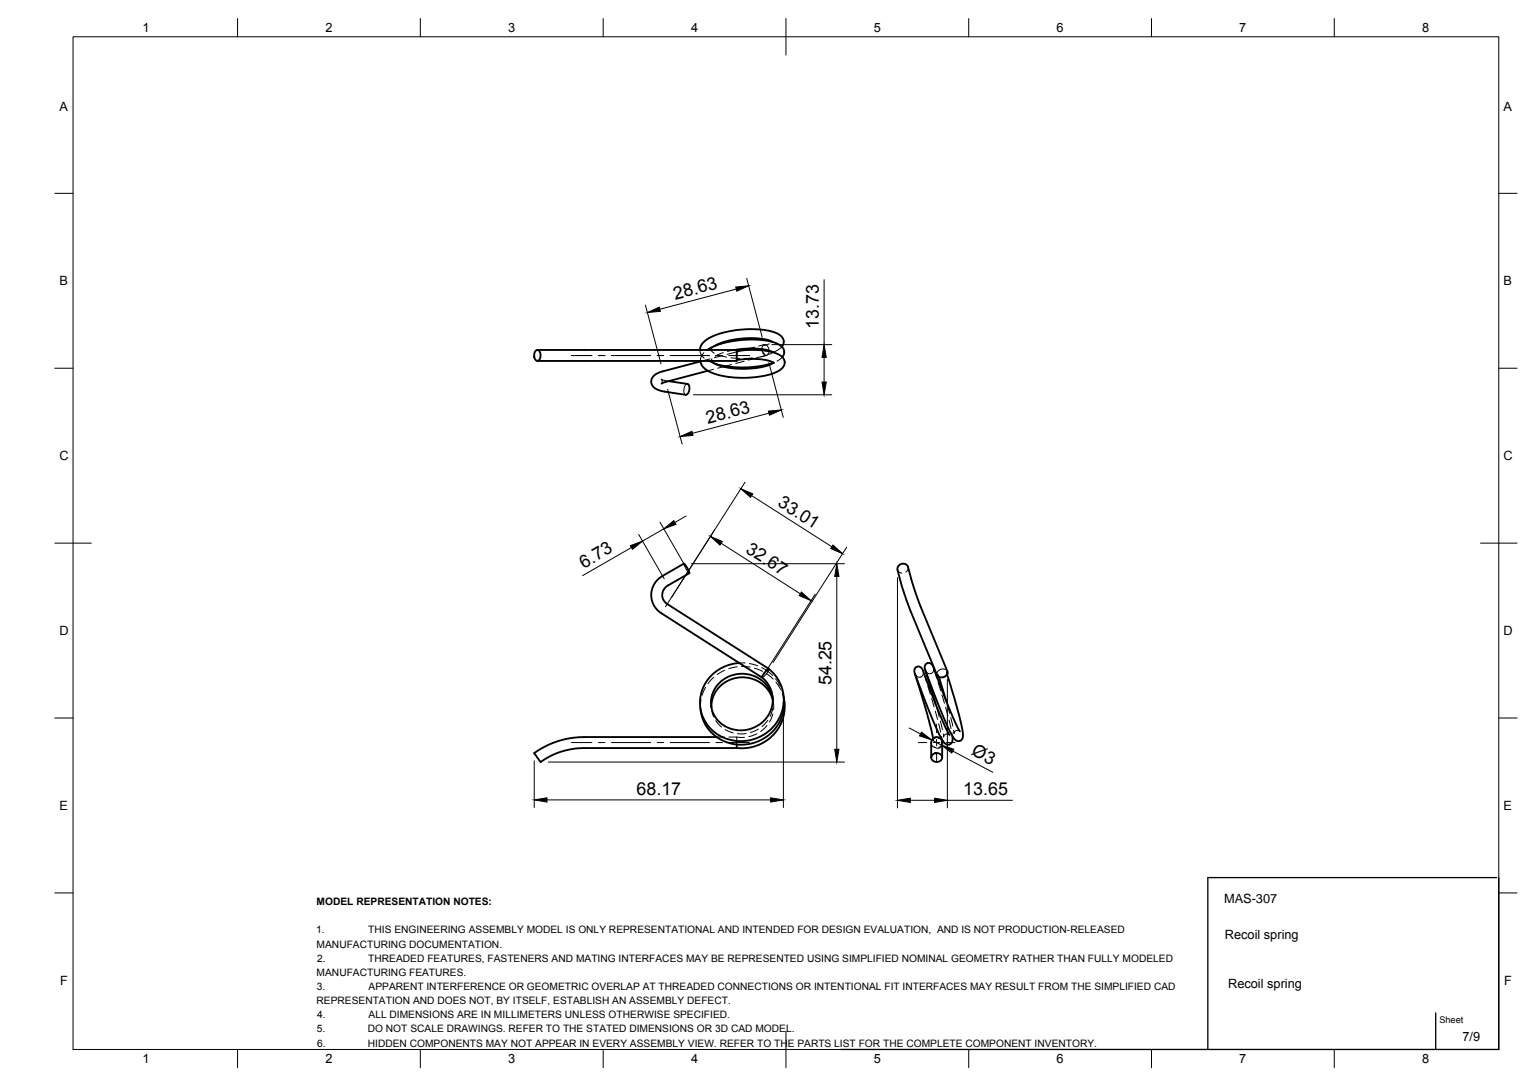
ISO-10303-21;
HEADER;
FILE_DESCRIPTION (('STEP AP214'),
    '1' );
FILE_NAME ('Recoil spring.step',
    '2026-10-06T07:34:29',
    ( '' ),
    ( '' ),
    'SwSTEP 2.0',
    'SolidWorks 2025',
    '' );
FILE_SCHEMA (( 'AUTOMOTIVE_DESIGN' ));
ENDSEC;

DATA;
#11=CARTESIAN_POINT ( 'NONE',  ( 205.4931693814993139, 33.91842896272902408, -6.501828201457912293 ) ) ;
#21=CARTESIAN_POINT ( 'NONE',  ( 205.4699394944333051, 33.88363592193200446, -7.930995773285529182 ) ) ;
#30=CARTESIAN_POINT ( 'NONE',  ( 198.8634854004546071, 49.55149448133588663, -6.680369717582868461 ) ) ;
#56=TOROIDAL_SURFACE ( 'NONE', #1821, 4.799128011492294732, 1.499999999999997113 ) ;
#64=CARTESIAN_POINT ( 'NONE',  ( 207.1592428330643827, 35.64176030267155681, -3.375779224823745928 ) ) ;
#71=CARTESIAN_POINT ( 'NONE',  ( 198.4684236769687686, 29.09143143995051872, -2.316743362709667409 ) ) ;
#88=CARTESIAN_POINT ( 'NONE',  ( 198.7876695280922661, 49.53587328158837977, -8.249370650301745655 ) ) ;
#95=CARTESIAN_POINT ( 'NONE',  ( 201.7406124912899941, 52.65652330452660834, -2.244206067705167396 ) ) ;
#103=CARTESIAN_POINT ( 'NONE',  ( 202.3883256910358739, 32.65987148549056229, -8.116337980372584582 ) ) ;
#123=DIRECTION ( 'NONE',  ( -0.9741547192086867923, 0.2258817899775114602, 0.000000000000000000 ) ) ;
#132=CARTESIAN_POINT ( 'NONE',  ( 202.9578473199472057, 32.84482942423175444, -9.656098271102047548 ) ) ;
#152=FACE_OUTER_BOUND ( 'NONE', #9575, .T. ) ;
#166=CARTESIAN_POINT ( 'NONE',  ( 198.3913412372077687, 29.09831693401786268, -0.7477385443502184703 ) ) ;
#174=CARTESIAN_POINT ( 'NONE',  ( 207.1690005588685040, 46.08364065960329725, 0.3832845883476674320 ) ) ;
#205=CARTESIAN_POINT ( 'NONE',  ( 205.4339596421060889, 33.86846485884471747, -4.932823326473320336 ) ) ;
#208=CIRCLE ( 'NONE', #2252, 1.499999999999996891 ) ;
#212=CARTESIAN_POINT ( 'NONE',  ( 192.9105869384611935, 31.39693960586098598, -5.567602151433582058 ) ) ;
#219=AXIS2_PLACEMENT_3D ( 'NONE', #7961, #12749, #6770 ) ;
#229=EDGE_CURVE ( 'NONE', #11059, #5257, #8156, .T. ) ;
#231=DIRECTION ( 'NONE',  ( 0.9296197478520974444, 0.3660421972118351741, -0.04266420354037655377 ) ) ;
#237=CARTESIAN_POINT ( 'NONE',  ( 207.1194509196011495, 46.14302886020001182, -1.185720282267065828 ) ) ;
#249=CARTESIAN_POINT ( 'NONE',  ( 194.7047954745769687, 33.92018974228710704, -0.9908858387024377379 ) ) ;
#258=CARTESIAN_POINT ( 'NONE',  ( 202.9147226314038051, 48.88641379461363101, -0.9068510277452211943 ) ) ;
#277=ORIENTED_EDGE ( 'NONE', *, *, #6163, .F. ) ;
#281=DIRECTION ( 'NONE',  ( -0.9741547192086869034, 0.2258817899775114879, 0.000000000000000000 ) ) ;
#291=CARTESIAN_POINT ( 'NONE',  ( 191.3844089520862894, 42.02011290432638901, -3.056456915890917170 ) ) ;
#298=CARTESIAN_POINT ( 'NONE',  ( 204.3096479244403554, 51.57035008254927533, -0.9325724660367167296 ) ) ;
#317=CARTESIAN_POINT ( 'NONE',  ( 207.1167095084715868, 46.15093117762712893, -7.185265714380067337 ) ) ;
#325=CARTESIAN_POINT ( 'NONE',  ( 203.1202131991386182, 29.73909689272393564, -6.555651296533415717 ) ) ;
#329=TOROIDAL_SURFACE ( 'NONE', #6419, 4.799128011492294732, 1.499999999999997113 ) ;
#334=CARTESIAN_POINT ( 'NONE',  ( 198.9393012728169765, 49.56711568108339350, -5.111368784863990378 ) ) ;
#366=CARTESIAN_POINT ( 'NONE',  ( 194.7957337413261030, 33.86335648926068842, -5.558215102112974648 ) ) ;
#393=CARTESIAN_POINT ( 'NONE',  ( 198.8872864542346974, 32.16591232847088122, -2.310211674251309688 ) ) ;
#410=CARTESIAN_POINT ( 'NONE',  ( 194.8975446553719451, 47.93174114899129989, -1.867390259657528251 ) ) ;
#442=CARTESIAN_POINT ( 'NONE',  ( 208.8124460758720033, 42.05191026284237665, -4.433604294307299298 ) ) ;
#471=CARTESIAN_POINT ( 'NONE',  ( 198.8863654052626657, 49.55881746625484396, -3.681704842056328086 ) ) ;
#489=CARTESIAN_POINT ( 'NONE',  ( 201.2644297667355886, 32.15691159195442594, -0.6119088838163699862 ) ) ;
#491=ADVANCED_FACE ( 'NONE', ( #11969 ), #1138, .F. ) ;
#494=DIRECTION ( 'NONE',  ( 0.000000000000000000, 0.9569673715906176215, 0.2901955370279575286 ) ) ;
#525=CARTESIAN_POINT ( 'NONE',  ( 207.1194509196011495, 46.14302886020001182, -1.185720282267065828 ) ) ;
#557=CARTESIAN_POINT ( 'NONE',  ( 205.4319281802536068, 33.87189768065903905, -1.932853472788024440 ) ) ;
#566=CARTESIAN_POINT ( 'NONE',  ( 202.1731860119849102, 31.08132011834958419, -8.150590381057213563 ) ) ;
#575=CARTESIAN_POINT ( 'NONE',  ( 207.3546231538492179, 50.29643094772573164, -2.498001438440778710 ) ) ;
#577=EDGE_LOOP ( 'NONE', ( #6152, #5245, #8146, #7504 ) ) ;
#580=LINE ( 'NONE', #12899, #7977 ) ;
#623=CARTESIAN_POINT ( 'NONE',  ( 203.1375244286944906, 48.81137831324044640, 0.6531691591918254991 ) ) ;
#642=MANIFOLD_SOLID_BREP ( 'Sweep1', #13662 ) ;
#651=CARTESIAN_POINT ( 'NONE',  ( 211.8663679066739007, 39.14335912920272875, 0.001962313962203070510 ) ) ;
#654=CARTESIAN_POINT ( 'NONE',  ( 166.7445055987502656, 66.43865443379107205, -0.9107274384406879308 ) ) ;
#688=DIRECTION ( 'NONE',  ( 0.6130913241491352528, 0.7900120431063440973, -6.390853288732736916E-17 ) ) ;
#690=PRODUCT ( 'Recoil spring', 'Recoil spring', '', ( #15067 ) ) ;
#693=FACE_OUTER_BOUND ( 'NONE', #15416, .T. ) ;
#706=DIRECTION ( 'NONE',  ( -1.000000000000000000, 0.000000000000000000, 0.000000000000000000 ) ) ;
#709=CARTESIAN_POINT ( 'NONE',  ( 205.5168546899054434, 47.82311440310952833, -1.064259200291542529 ) ) ;
#724=EDGE_LOOP ( 'NONE', ( #6088, #7663, #14419, #15071, #11022 ) ) ;
#727=CARTESIAN_POINT ( 'NONE',  ( 201.6516474359912934, 52.64960446646696113, -8.385050746608255778 ) ) ;
#736=VECTOR ( 'NONE', #8355, 999.9999999999998863 ) ;
#780=CARTESIAN_POINT ( 'NONE',  ( 207.3736904795575811, 50.31851200600168994, -2.642755332960478043 ) ) ;
#790=DIRECTION ( 'NONE',  ( -1.000000000000000000, 0.000000000000000000, 0.000000000000000000 ) ) ;
#809=CARTESIAN_POINT ( 'NONE',  ( 188.2965488188713721, 39.35787245461563089, -4.374714073396582137 ) ) ;
#863=CARTESIAN_POINT ( 'NONE',  ( 198.5781842723177704, 29.07471546161169229, -6.884323831650920766 ) ) ;
#870=DIRECTION ( 'NONE',  ( 0.000000000000000000, 0.000000000000000000, -1.000000000000000000 ) ) ;
#887=CARTESIAN_POINT ( 'NONE',  ( 190.6753907620029054, 48.10438271498464502, -4.747728522856008659 ) ) ;
#898=CARTESIAN_POINT ( 'NONE',  ( 208.8119045081773777, 39.60750423734790360, -5.989029428842635561 ) ) ;
#906=TOROIDAL_SURFACE ( 'NONE', #7237, 21.91351791792154202, 1.499999999999997113 ) ;
#965=CARTESIAN_POINT ( 'NONE',  ( 198.8104769829885754, 49.54338459298288200, -5.250705761417654216 ) ) ;
#975=CARTESIAN_POINT ( 'NONE',  ( 198.8872864542346974, 32.16591232847088122, -2.310211674251309688 ) ) ;
#982=CIRCLE ( 'NONE', #8569, 1.499999999999994227 ) ;
#983=CARTESIAN_POINT ( 'NONE',  ( 208.8060099514817978, 42.07246638764446089, -7.432400171711813996 ) ) ;
#996=DIRECTION ( 'NONE',  ( 0.000000000000000000, 0.000000000000000000, -1.000000000000000000 ) ) ;
#1021=CARTESIAN_POINT ( 'NONE',  ( 192.9079700310636269, 50.30505391962363149, -5.011923969639807019 ) ) ;
#1022=PRESENTATION_STYLE_ASSIGNMENT (( #8312 ) ) ;
#1052=CARTESIAN_POINT ( 'NONE',  ( 207.1558710170397433, 35.63411313097393673, -9.376170956558697256 ) ) ;
#1063=CARTESIAN_POINT ( 'NONE',  ( 201.2541767070109984, 32.14103196098812987, -5.186035738131804962 ) ) ;
#1081=FACE_OUTER_BOUND ( 'NONE', #6812, .T. ) ;
#1088=SHAPE_REPRESENTATION_RELATIONSHIP ( 'NONE' , 'NONE' ,  #5419, #10743 ) ;
#1097=EDGE_CURVE ( 'NONE', #8873, #8651, #1552, .T. ) ;
#1100=CARTESIAN_POINT ( 'NONE',  ( 208.8060099514817978, 42.07246638764446089, -7.432400171711813996 ) ) ;
#1102=EDGE_LOOP ( 'NONE', ( #10073, #2655 ) ) ;
#1128=CARTESIAN_POINT ( 'NONE',  ( 211.8745662956760896, 42.53653439883859022, -6.011979689023970508 ) ) ;
#1130=CARTESIAN_POINT ( 'NONE',  ( 166.9217645774054120, 62.57671370024034729, -0.9107274384406883749 ) ) ;
#1136=CARTESIAN_POINT ( 'NONE',  ( 198.8634854004546071, 49.55149448133588663, -6.680369717582868461 ) ) ;
#1138=PLANE ( 'NONE',  #4834 ) ;
#1145=CARTESIAN_POINT ( 'NONE',  ( 208.8051451104704768, 39.65587490144260840, -4.559632177755815086 ) ) ;
#1172=CARTESIAN_POINT ( 'NONE',  ( 205.4931693814993139, 33.91842896272902408, -6.501828201457912293 ) ) ;
#1186=ORIENTED_EDGE ( 'NONE', *, *, #3880, .F. ) ;
#1195=CARTESIAN_POINT ( 'NONE',  ( 211.8802283582561472, 39.29745248741442509, -3.136047433260559902 ) ) ;
#1208=CARTESIAN_POINT ( 'NONE',  ( 198.8863654052626657, 49.55881746625484396, -3.681704842056328086 ) ) ;
#1216=CARTESIAN_POINT ( 'NONE',  ( 201.2541767070109984, 32.14103196098812987, -5.186035738131804962 ) ) ;
#1231=DIRECTION ( 'NONE',  ( -0.2258817899775119320, -0.9741547192086866813, 0.000000000000000000 ) ) ;
#1255=CARTESIAN_POINT ( 'NONE',  ( 198.9643688939780191, 32.15902683440354082, -3.879216492611309519 ) ) ;
#1261=CARTESIAN_POINT ( 'NONE',  ( 192.9009781015629699, 50.32399521507879570, -6.439879401016198379 ) ) ;
#1282=CARTESIAN_POINT ( 'NONE',  ( 201.1886137893777970, 49.58779752487713210, -5.375724496774349603 ) ) ;
#1290=EDGE_CURVE ( 'NONE', #2155, #10688, #5789, .T. ) ;
#1291=CARTESIAN_POINT ( 'NONE',  ( 209.6520103264654438, 47.93571987055528183, -2.624305162434556582 ) ) ;
#1292=ORIENTED_EDGE ( 'NONE', *, *, #10887, .T. ) ;
#1320=ORIENTED_EDGE ( 'NONE', *, *, #15180, .T. ) ;
#1331=CARTESIAN_POINT ( 'NONE',  ( 208.8253499713366352, 39.76173270276598970, -9.127040822819912691 ) ) ;
#1356=CARTESIAN_POINT ( 'NONE',  ( 205.5168546899054434, 47.82311440310952833, -1.064259200291542529 ) ) ;
#1366=CARTESIAN_POINT ( 'NONE',  ( 190.5757627275658876, 33.76246512414177658, -1.122914728280356433 ) ) ;
#1371=CARTESIAN_POINT ( 'NONE',  ( 170.6931741512129577, -3.595212766542494887, -13.46247879130521952 ) ) ;
#1374=CARTESIAN_POINT ( 'NONE',  ( 201.3430548014149792, 49.57506994421799362, -2.237714600605053228 ) ) ;
#1386=CARTESIAN_POINT ( 'NONE',  ( 169.1145417280692698, 64.59938046134368506, -0.9107274384406877088 ) ) ;
#1392=LINE ( 'NONE', #3931, #8028 ) ;
#1403=EDGE_CURVE ( 'NONE', #5373, #11059, #4546, .T. ) ;
#1406=CARTESIAN_POINT ( 'NONE',  ( 194.7298858349713271, 47.80990288192585780, -8.002378029496236778 ) ) ;
#1413=CARTESIAN_POINT ( 'NONE',  ( 209.5813200025016840, 33.68906342850529256, -7.816773541869418196 ) ) ;
#1415=EDGE_CURVE ( 'NONE', #11153, #5773, #6043, .T. ) ;
#1421=ORIENTED_EDGE ( 'NONE', *, *, #1403, .T. ) ;
#1433=CARTESIAN_POINT ( 'NONE',  ( 193.1265229109121435, 35.50728864820005981, -5.680987958736793075 ) ) ;
#1439=CARTESIAN_POINT ( 'NONE',  ( 191.3907470605235801, 42.09736693221333326, -1.487451979171016125 ) ) ;
#1449=CARTESIAN_POINT ( 'NONE',  ( 205.4081958545874613, 47.87064854543508829, -4.057643371672452481 ) ) ;
#1485=CARTESIAN_POINT ( 'NONE',  ( 191.3918663844754349, 39.68659111044760124, -5.934329888686073140 ) ) ;
#1493=CARTESIAN_POINT ( 'NONE',  ( 190.6654829352982290, 48.12161981134465805, -3.320406740534335377 ) ) ;
#1517=CARTESIAN_POINT ( 'NONE',  ( 207.1288103955774318, 46.12660085639766550, -4.186765234109192768 ) ) ;
#1527=CARTESIAN_POINT ( 'NONE',  ( 188.2965488188713721, 39.35787245461563089, -4.374714073396582137 ) ) ;
#1535=CARTESIAN_POINT ( 'NONE',  ( 198.9622538275367845, 49.57425033952682014, -2.112703922695001513 ) ) ;
#1552=LINE ( 'NONE', #13232, #4560 ) ;
#1595=CARTESIAN_POINT ( 'NONE',  ( 191.3844089520862894, 42.02011290432638901, -3.056456915890917170 ) ) ;
#1603=EDGE_CURVE ( 'NONE', #11059, #9376, #6576, .T. ) ;
#1618=CARTESIAN_POINT ( 'NONE',  ( 191.3767946852191528, 39.76267059705192253, -4.365329018565075714 ) ) ;
#1675=CARTESIAN_POINT ( 'NONE',  ( 198.8863654052626657, 49.55881746625484396, -3.681704842056328086 ) ) ;
#1676=ORIENTED_EDGE ( 'NONE', *, *, #12956, .T. ) ;
#1685=DIRECTION ( 'NONE',  ( -0.8204839007831801201, 0.5707893219124390294, -0.03171306586179811760 ) ) ;
#1692=CARTESIAN_POINT ( 'NONE',  ( 194.7047954745769687, 33.92018974228710704, -0.9908858387024377379 ) ) ;
#1740=ORIENTED_EDGE ( 'NONE', *, *, #9984, .T. ) ;
#1752=CARTESIAN_POINT ( 'NONE',  ( 193.1249951165660548, 46.22013307728793308, -3.310989833511668756 ) ) ;
#1754=DIRECTION ( 'NONE',  ( -0.2258817899775119320, -0.9741547192086866813, 0.000000000000000000 ) ) ;
#1771=CARTESIAN_POINT ( 'NONE',  ( 207.2666510146856069, 31.35441966018789728, -3.370316356820458381 ) ) ;
#1803=CARTESIAN_POINT ( 'NONE',  ( 191.4227524587821279, 39.61567282607229856, -2.929995994935606252 ) ) ;
#1810=DIRECTION ( 'NONE',  ( -0.7900120431063429871, 0.6130913241491365850, 0.000000000000000000 ) ) ;
#1811=CARTESIAN_POINT ( 'NONE',  ( 173.2749560924322907, 69.96037208313981637, -0.9107274384406881529 ) ) ;
#1818=CARTESIAN_POINT ( 'NONE',  ( 207.3157014670556748, 31.37515976295564357, -6.367693553816072161 ) ) ;
#1821=AXIS2_PLACEMENT_3D ( 'NONE', #5536, #6883, #15294 ) ;
#1844=CARTESIAN_POINT ( 'NONE',  ( 198.4239224672526234, 29.08807987246144933, -3.746314016867685837 ) ) ;
#1851=DIRECTION ( 'NONE',  ( 0.000000000000000000, 0.9569673715906176215, 0.2901955370279575286 ) ) ;
#1892=CARTESIAN_POINT ( 'NONE',  ( 201.6895650671498288, 29.08490409614774208, -0.6212496039192949571 ) ) ;
#1901=EDGE_LOOP ( 'NONE', ( #1292, #1740, #6793, #7476 ) ) ;
#1906=CARTESIAN_POINT ( 'NONE',  ( 205.4339596421060889, 33.86846485884471747, -4.932823326473320336 ) ) ;
#1921=CARTESIAN_POINT ( 'NONE',  ( 209.6393851568315938, 47.95822392590527983, 0.3767681043515945238 ) ) ;
#1957=FACE_OUTER_BOUND ( 'NONE', #577, .T. ) ;
#1960=LINE ( 'NONE', #6798, #8102 ) ;
#1970=CARTESIAN_POINT ( 'NONE',  ( 207.2819921120892275, 50.35227183911742088, -8.638656677529437999 ) ) ;
#1979=DIRECTION ( 'NONE',  ( 0.000000000000000000, 0.000000000000000000, -1.000000000000000000 ) ) ;
#1999=CARTESIAN_POINT ( 'NONE',  ( 198.5423134874356208, 52.64753739496011065, -2.122073255223759780 ) ) ;
#2041=DIRECTION ( 'NONE',  ( 0.000000000000000000, 0.000000000000000000, -1.000000000000000000 ) ) ;
#2050=CARTESIAN_POINT ( 'NONE',  ( 207.5020891771285960, 50.23084475345794431, 0.4952462535581279024 ) ) ;
#2080=CARTESIAN_POINT ( 'NONE',  ( 207.2638851143210275, 31.35908548908414417, -0.3703513705075706097 ) ) ;
#2130=CARTESIAN_POINT ( 'NONE',  ( 188.3492591927541753, 42.47468418338397811, -7.638025320682917396 ) ) ;
#2146=ORIENTED_EDGE ( 'NONE', *, *, #4376, .F. ) ;
#2155=VERTEX_POINT ( 'NONE', #1811 ) ;
#2157=CARTESIAN_POINT ( 'NONE',  ( 194.7298858349713271, 47.80990288192585780, -8.002378029496236778 ) ) ;
#2170=CARTESIAN_POINT ( 'NONE',  ( 191.4249991583111523, 42.11970308376083949, -6.062475933048471433 ) ) ;
#2211=CARTESIAN_POINT ( 'NONE',  ( 203.2625657313046190, 29.78760669494945645, -9.693656633365744568 ) ) ;
#2236=CARTESIAN_POINT ( 'NONE',  ( 193.0816233526163046, 46.15577860858359571, -4.879990690958216248 ) ) ;
#2248=CARTESIAN_POINT ( 'NONE',  ( 207.0703735592109069, 35.50494473061488065, -6.238171316985951620 ) ) ;
#2252=AXIS2_PLACEMENT_3D ( 'NONE', #1130, #15560, #8420 ) ;
#2256=CARTESIAN_POINT ( 'NONE',  ( 198.9111841706756536, 32.15857605477618364, -5.308824953579920347 ) ) ;
#2277=CIRCLE ( 'NONE', #12605, 23.41351791792154202 ) ;
#2280=CARTESIAN_POINT ( 'NONE',  ( 202.9928097691983169, 48.86380790798758511, -0.9029304599467440351 ) ) ;
#2291=CARTESIAN_POINT ( 'NONE',  ( 205.4699394944333051, 33.88363592193200446, -7.930995773285529182 ) ) ;
#2301=ORIENTED_EDGE ( 'NONE', *, *, #12956, .F. ) ;
#2321=CARTESIAN_POINT ( 'NONE',  ( 193.1767286061335653, 35.44822858574072910, -7.249992917093472933 ) ) ;
#2332=CARTESIAN_POINT ( 'NONE',  ( 191.3918663844754349, 39.68659111044760124, -5.934329888686073140 ) ) ;
#2341=CARTESIAN_POINT ( 'NONE',  ( 207.1131222881253393, 35.56952893079440514, -7.807171136772324438 ) ) ;
#2370=CARTESIAN_POINT ( 'NONE',  ( 207.1558710170397433, 35.63411313097393673, -9.376170956558697256 ) ) ;
#2388=EDGE_CURVE ( 'NONE', #6288, #10688, #1960, .T. ) ;
#2397=CARTESIAN_POINT ( 'NONE',  ( 198.3905366428873549, 52.61667164843417765, -5.260075093946414704 ) ) ;
#2406=CARTESIAN_POINT ( 'NONE',  ( 201.3402840685550643, 32.17245832385849980, -2.180909807981465054 ) ) ;
#2447=CARTESIAN_POINT ( 'NONE',  ( 205.5291621427655002, 33.93354315402728361, -9.500001906449378808 ) ) ;
#2470=CARTESIAN_POINT ( 'NONE',  ( 205.4911088677281725, 33.92184391926740972, -3.501858402168778639 ) ) ;
#2484=CARTESIAN_POINT ( 'NONE',  ( 198.4239224672526234, 29.08807987246144933, -3.746314016867685837 ) ) ;
#2489=DIRECTION ( 'NONE',  ( -0.1562424607007877608, 0.2866315678550999668, -0.9452145987991775744 ) ) ;
#2528=CARTESIAN_POINT ( 'NONE',  ( 202.4595012533446550, 32.68412682837883665, -9.685340726858029825 ) ) ;
#2535=CARTESIAN_POINT ( 'NONE',  ( 209.5863484626195543, 33.70058422559537092, -1.816147585399736863 ) ) ;
#2552=CIRCLE ( 'NONE', #3062, 3.299128011492291623 ) ;
#2566=CARTESIAN_POINT ( 'NONE',  ( 190.7088546992480076, 48.18597428004899541, -1.751405883087224113 ) ) ;
#2608=CARTESIAN_POINT ( 'NONE',  ( 202.3883256910358739, 32.65987148549056229, -8.116337980372584582 ) ) ;
#2635=CARTESIAN_POINT ( 'NONE',  ( 194.7691866843436799, 33.87697957786221536, -2.559886773443665220 ) ) ;
#2645=CARTESIAN_POINT ( 'NONE',  ( 198.5110307061451067, 52.63772278181842523, -5.120705508804510586 ) ) ;
#2653=CARTESIAN_POINT ( 'NONE',  ( 203.1375244286944906, 48.81137831324044640, 0.6531691591918254991 ) ) ;
#2655=ORIENTED_EDGE ( 'NONE', *, *, #1415, .F. ) ;
#2712=CARTESIAN_POINT ( 'NONE',  ( 208.8124460758720033, 42.05191026284237665, -4.433604294307299298 ) ) ;
#2720=CARTESIAN_POINT ( 'NONE',  ( 193.1683668805158334, 46.28448754599228465, -1.741988976065122152 ) ) ;
#2730=CARTESIAN_POINT ( 'NONE',  ( 191.4227524587821279, 39.61567282607229856, -2.929995994935606252 ) ) ;
#2773=CARTESIAN_POINT ( 'NONE',  ( 188.3535365708562779, 39.18556319200014570, -2.939344140512093251 ) ) ;
#2774=CIRCLE ( 'NONE', #11846, 1.499999999999988232 ) ;
#2780=ORIENTED_EDGE ( 'NONE', *, *, #4665, .F. ) ;
#2785=CYLINDRICAL_SURFACE ( 'NONE', #15558, 1.500000000000000444 ) ;
#2792=LINE ( 'NONE', #7617, #5517 ) ;
#2793=CARTESIAN_POINT ( 'NONE',  ( 202.9147226314038051, 48.88641379461363101, -0.9068510277452211943 ) ) ;
#2813=CARTESIAN_POINT ( 'NONE',  ( 202.8187013049204950, 32.78779105710274422, -6.518094968334741779 ) ) ;
#2852=CARTESIAN_POINT ( 'NONE',  ( 209.6082252582704371, 33.74895655718308518, -4.813932606105665535 ) ) ;
#2869=FACE_OUTER_BOUND ( 'NONE', #5166, .T. ) ;
#2873=CARTESIAN_POINT ( 'NONE',  ( 203.1427736312160164, 48.80054947466439330, -2.493724563924679671 ) ) ;
#2884=ORIENTED_EDGE ( 'NONE', *, *, #4665, .T. ) ;
#2892=CARTESIAN_POINT ( 'NONE',  ( 208.8213467238098247, 41.99652926550911758, -5.863399402755005596 ) ) ;
#2909=AXIS2_PLACEMENT_3D ( 'NONE', #7942, #5322, #5486 ) ;
#2923=CARTESIAN_POINT ( 'NONE',  ( 208.8002188652075972, 39.64064887424692785, -1.560527519332197022 ) ) ;
#2964=UNCERTAINTY_MEASURE_WITH_UNIT (LENGTH_MEASURE( 1.000000000000000082E-05 ), #13235, 'distance_accuracy_value', 'NONE');
#2965=CARTESIAN_POINT ( 'NONE',  ( 208.8276044750562335, 41.97590694738037342, -2.864603354092789100 ) ) ;
#2997=CARTESIAN_POINT ( 'NONE',  ( 194.7891036845171300, 47.85977741052224133, -6.433373108600371815 ) ) ;
#3015=CARTESIAN_POINT ( 'NONE',  ( 192.9601959511087728, 50.37386974367067438, -4.870874480120333416 ) ) ;
#3027=CARTESIAN_POINT ( 'NONE',  ( 205.4496313998743915, 47.84832575209421890, -7.060263518810960370 ) ) ;
#3045=CARTESIAN_POINT ( 'NONE',  ( 202.5558682508970492, 29.63341987102701580, -9.723657537314917221 ) ) ;
#3046=ORIENTED_EDGE ( 'NONE', *, *, #1403, .F. ) ;
#3054=ADVANCED_FACE ( 'NONE', ( #9769 ), #906, .T. ) ;
#3062=AXIS2_PLACEMENT_3D ( 'NONE', #5627, #1979, #706 ) ;
#3094=CARTESIAN_POINT ( 'NONE',  ( 204.3809113867051508, 51.54681031777401756, 0.6364305089822913652 ) ) ;
#3112=ORIENTED_EDGE ( 'NONE', *, *, #6453, .T. ) ;
#3118=CARTESIAN_POINT ( 'NONE',  ( 192.8103048780560584, 31.45858264101640600, -1.000270116828862133 ) ) ;
#3165=CARTESIAN_POINT ( 'NONE',  ( 198.3905366428873549, 52.61667164843417765, -5.260075093946414704 ) ) ;
#3176=CARTESIAN_POINT ( 'NONE',  ( 208.8162124854775357, 42.04914431719598156, -1.433821094984975009 ) ) ;
#3183=EDGE_CURVE ( 'NONE', #10985, #5154, #580, .T. ) ;
#3189=DIRECTION ( 'NONE',  ( -0.9429519417310716634, 0.3294944882152614496, 0.04769714688914629408 ) ) ;
#3192=CARTESIAN_POINT ( 'NONE',  ( 198.5781842723177704, 29.07471546161169229, -6.884323831650920766 ) ) ;
#3227=CARTESIAN_POINT ( 'NONE',  ( 172.0899380277727744, 70.88000906936352408, -0.9107274384406883749 ) ) ;
#3236=ORIENTED_EDGE ( 'NONE', *, *, #1603, .T. ) ;
#3238=CARTESIAN_POINT ( 'NONE',  ( 207.2638851143210275, 31.35908548908414417, -0.3703513705075706097 ) ) ;
#3270=CARTESIAN_POINT ( 'NONE',  ( 207.3157014670556748, 31.37515976295564357, -6.367693553816072161 ) ) ;
#3322=CARTESIAN_POINT ( 'NONE',  ( 211.8657363685815653, 42.56416725473636831, -9.010781945348840694 ) ) ;
#3350=CARTESIAN_POINT ( 'NONE',  ( 198.5455061167297117, 29.08454594588317477, -3.885748181069116569 ) ) ;
#3358=AXIS2_PLACEMENT_3D ( 'NONE', #4025, #688, #1810 ) ;
#3361=CARTESIAN_POINT ( 'NONE',  ( 208.8213467238098247, 41.99652926550911758, -5.863399402755005596 ) ) ;
#3400=CARTESIAN_POINT ( 'NONE',  ( 192.9750851430037528, 31.35397111148814631, -7.136603044727629630 ) ) ;
#3427=CARTESIAN_POINT ( 'NONE',  ( 208.7906731791537425, 42.14840350977979710, -9.001400940668622397 ) ) ;
#3436=CARTESIAN_POINT ( 'NONE',  ( 208.8051451104704768, 39.65587490144260840, -4.559632177755815086 ) ) ;
#3446=CARTESIAN_POINT ( 'NONE',  ( 205.4496313998743915, 47.84832575209421890, -7.060263518810960370 ) ) ;
#3450=CARTESIAN_POINT ( 'NONE',  ( 202.3883256910358739, 32.65987148549056229, -8.116337980372584582 ) ) ;
#3473=CARTESIAN_POINT ( 'NONE',  ( 201.4161383703745400, 32.18800505576257365, -3.749910732146560122 ) ) ;
#3501=CARTESIAN_POINT ( 'NONE',  ( 201.8412736707888087, 29.11599755995149152, -3.759251452247287517 ) ) ;
#3512=CARTESIAN_POINT ( 'NONE',  ( 202.3883256910358739, 32.65987148549056229, -8.116337980372584582 ) ) ;
#3518=CARTESIAN_POINT ( 'NONE',  ( 203.7481738146713326, 51.76374178194004827, -0.9107274384406881529 ) ) ;
#3521=APPLICATION_CONTEXT ( 'automotive_design' ) ;
#3555=CARTESIAN_POINT ( 'NONE',  ( 205.4496313998743915, 47.84832575209421890, -7.060263518810960370 ) ) ;
#3569=COLOUR_RGB ( '', 0.40784314, 0.44705882, 0.49803922) ;
#3583=CARTESIAN_POINT ( 'NONE',  ( 209.5402858782260864, 48.07700032709870896, -2.761241636875660710 ) ) ;
#3593=CARTESIAN_POINT ( 'NONE',  ( 201.8629198063431716, 32.54887535240757757, -8.146526315903498627 ) ) ;
#3602=FACE_OUTER_BOUND ( 'NONE', #11632, .T. ) ;
#3623=DIRECTION ( 'NONE',  ( -1.000000000000000000, 0.000000000000000000, 0.000000000000000000 ) ) ;
#3634=AXIS2_PLACEMENT_3D ( 'NONE', #14195, #11917, #9474 ) ;
#3642=CARTESIAN_POINT ( 'NONE',  ( 201.7746181419471725, 32.40197136543856971, -7.616432591815856412 ) ) ;
#3653=ORIENTED_EDGE ( 'NONE', *, *, #10887, .F. ) ;
#3656=CARTESIAN_POINT ( 'NONE',  ( 205.3436520073863107, 47.91354567463725544, -5.626644267508417840 ) ) ;
#3666=CARTESIAN_POINT ( 'NONE',  ( 205.4107168461011099, 33.83372868983673243, -6.361989640121679557 ) ) ;
#3690=ORIENTED_EDGE ( 'NONE', *, *, #8722, .T. ) ;
#3707=CARTESIAN_POINT ( 'NONE',  ( 194.7786688470199010, 47.83282381504752578, -5.005399988216014506 ) ) ;
#3713=CARTESIAN_POINT ( 'NONE',  ( 207.3230658017955932, 31.40903172769477081, -1.939356299889454016 ) ) ;
#3718=DIRECTION ( 'NONE',  ( -0.3662838836490099337, 0.9305003370641709015, 0.002288952263120960697 ) ) ;
#3739=DIRECTION ( 'NONE',  ( 0.5602235199536453880, 0.8138631617988981715, 0.1541958545404129299 ) ) ;
#3746=CARTESIAN_POINT ( 'NONE',  ( 193.0268458394156710, 50.40397125358524733, -1.873914241081319210 ) ) ;
#3791=CARTESIAN_POINT ( 'NONE',  ( 208.8010691282704840, 42.12517885095529380, -3.002821972062079681 ) ) ;
#3797=CARTESIAN_POINT ( 'NONE',  ( 201.7287634318787752, 52.64281578357326907, -6.816045903392632610 ) ) ;
#3805=CIRCLE ( 'NONE', #13115, 1.499999999999996891 ) ;
#3819=CARTESIAN_POINT ( 'NONE',  ( 191.4249991583111523, 42.11970308376083949, -6.062475933048471433 ) ) ;
#3831=CARTESIAN_POINT ( 'NONE',  ( 193.0763172156907501, 35.56634871065938341, -4.111983000380113218 ) ) ;
#3839=CARTESIAN_POINT ( 'NONE',  ( 208.7932886394164598, 39.56360219514107257, 0.008477354278063056400 ) ) ;
#3860=CYLINDRICAL_SURFACE ( 'NONE', #10644, 1.499999999999995115 ) ;
#3875=CARTESIAN_POINT ( 'NONE',  ( 198.5010533697851827, 29.08139766703656903, -5.315318924259303301 ) ) ;
#3880=EDGE_CURVE ( 'NONE', #14252, #2155, #2792, .T. ) ;
#3902=CARTESIAN_POINT ( 'NONE',  ( 203.7958462291278749, 29.94547861640233322, -6.526400227122580944 ) ) ;
#3910=CARTESIAN_POINT ( 'NONE',  ( 205.4107168461011099, 33.83372868983673243, -6.361989640121679557 ) ) ;
#3931=CARTESIAN_POINT ( 'NONE',  ( 203.0705284447388124, 48.84127762431399589, -0.9107274384406883749 ) ) ;
#3942=CARTESIAN_POINT ( 'NONE',  ( 201.3402840685550643, 32.17245832385849980, -2.180909807981465054 ) ) ;
#3952=EDGE_CURVE ( 'NONE', #9376, #7692, #15563, .T. ) ;
#3963=CARTESIAN_POINT ( 'NONE',  ( 201.3402840685550643, 32.17245832385849980, -2.180909807981465054 ) ) ;
#3964=ORIENTED_EDGE ( 'NONE', *, *, #3183, .T. ) ;
#3978=CARTESIAN_POINT ( 'NONE',  ( 193.0763172156907501, 35.56634871065938341, -4.111983000380113218 ) ) ;
#3984=DIRECTION ( 'NONE',  ( -0.1562424607007877608, 0.2866315678550999668, -0.9452145987991775744 ) ) ;
#4012=CARTESIAN_POINT ( 'NONE',  ( 191.4249991583111523, 42.11970308376083949, -6.062475933048471433 ) ) ;
#4025=CARTESIAN_POINT ( 'NONE',  ( 167.9295236634097819, 65.51901744756737855, -0.9107274384406879308 ) ) ;
#4044=CARTESIAN_POINT ( 'NONE',  ( 198.8872864542346974, 32.16591232847088122, -2.310211674251309688 ) ) ;
#4061=CARTESIAN_POINT ( 'NONE',  ( 198.8102040144913758, 32.17279782253822162, -0.7412068558913099681 ) ) ;
#4121=CARTESIAN_POINT ( 'NONE',  ( 208.8060099514817978, 42.07246638764446089, -7.432400171711813996 ) ) ;
#4135=CARTESIAN_POINT ( 'NONE',  ( 207.1288103955774318, 46.12660085639766550, -4.186765234109192768 ) ) ;
#4165=CARTESIAN_POINT ( 'NONE',  ( 203.0658429208174880, 48.83360436048501896, -0.9158339742359169477 ) ) ;
#4181=CARTESIAN_POINT ( 'NONE',  ( 208.7932886394164598, 39.56360219514107257, 0.008477354278063056400 ) ) ;
#4182=FACE_OUTER_BOUND ( 'NONE', #12272, .T. ) ;
#4192=CARTESIAN_POINT ( 'NONE',  ( 201.3402840685550643, 32.17245832385849980, -2.180909807981465054 ) ) ;
#4209=CARTESIAN_POINT ( 'NONE',  ( 190.5757627275658876, 33.76246512414177658, -1.122914728280356433 ) ) ;
#4229=ORIENTED_EDGE ( 'NONE', *, *, #229, .F. ) ;
#4258=CARTESIAN_POINT ( 'NONE',  ( 207.0737247153217311, 35.51262227952910422, -0.2377773810599485560 ) ) ;
#4270=CARTESIAN_POINT ( 'NONE',  ( 193.1265229109121435, 35.50728864820005981, -5.680987958736793075 ) ) ;
#4272=AXIS2_PLACEMENT_3D ( 'NONE', #14169, #8277, #12828 ) ;
#4289=CARTESIAN_POINT ( 'NONE',  ( 192.8460887339186343, 31.43990810023382920, -3.998601258139535819 ) ) ;
#4343=CARTESIAN_POINT ( 'NONE',  ( 188.2949840871649485, 42.33905491644829766, -4.631930676406226688 ) ) ;
#4354=CARTESIAN_POINT ( 'NONE',  ( 191.4249991583111523, 42.11970308376083949, -6.062475933048471433 ) ) ;
#4358=DIRECTION ( 'NONE',  ( -1.000000000000000000, 0.000000000000000000, 0.000000000000000000 ) ) ;
#4369=CARTESIAN_POINT ( 'NONE',  ( 211.9048830940805885, 42.38452776791458376, -2.873977808594950112 ) ) ;
#4372=CIRCLE ( 'NONE', #13186, 1.499999999999997558 ) ;
#4376=EDGE_CURVE ( 'NONE', #10688, #2155, #9061, .T. ) ;
#4419=CARTESIAN_POINT ( 'NONE',  ( 203.8319104552679448, 51.73948369304471839, -2.483607112462900446 ) ) ;
#4446=CARTESIAN_POINT ( 'NONE',  ( 198.5110307061451067, 52.63772278181842523, -5.120705508804510586 ) ) ;
#4471=DIRECTION ( 'NONE',  ( -0.9429519417310716634, 0.3294944882152614496, 0.04769714688914629408 ) ) ;
#4490=B_SPLINE_SURFACE_WITH_KNOTS ( 'NONE', 3, 3, ( 
 ( #3593, #3512, #4617, #21, #8349, #9445, #5806, #4541, #8428, #12979, #1136, #14241, #5885, #2170, #2332, #6999, #7163, #10704, #1063, #12035, #4693, #3436, #9515, #14395, #8500, #13208, #1208, #11735, #8270, #13046, #4859, #5963, #9677, #975, #2406, #4774, #13130, #6044, #7240, #14163, #10867, #11967, #9599, #15496 ),
 ( #14471, #14314, #10782, #3666, #2248, #898, #3361, #7082, #11888, #15568, #5729, #10542, #15337, #8200, #11810, #3831, #8574, #12112, #11463, #11174, #5165, #8650, #6123, #7466, #12261, #9913, #13519, #13368, #2720, #1439, #6279, #7846, #249, #14633, #5090, #9994, #4258, #4181, #12633, #13282, #13445, #5014, #623, #12341 ),
 ( #9020, #325, #3902, #1818, #14992, #4935, #5463, #7545, #13814, #11094, #2645, #3015, #10274, #14703, #1527, #15069, #11015, #2484, #14544, #8725, #9837, #6363, #7316, #1291, #10943, #95, #9755, #3746, #2566, #7396, #12186, #1366, #6204, #166, #1892, #3238, #8080, #5693, #7922, #12865, #2050, #3094, #9254, #13901 ),
 ( #13014, #2211, #12781, #6888, #12706, #9402, #3322, #6732, #1970, #5541, #9101, #9180, #11535, #2130, #8160, #11852, #3400, #863, #15298, #6964, #4496, #10354, #9330, #12942, #15149, #14047, #3165, #1021, #13979, #4343, #11619, #11772, #7997, #6807, #15226, #10588, #5617, #14202, #5847, #10666, #780, #15458, #10435, #4419 ),
 ( #7279, #2528, #132, #2447, #2370, #1331, #4733, #9641, #9481, #11054, #7433, #1406, #8465, #5921, #10745, #4820, #15530, #10828, #10983, #1172, #13170, #6239, #8536, #12076, #6004, #4654, #9558, #3707, #4975, #14589, #14277, #6091, #10908, #1255, #3473, #14436, #64, #13327, #3791, #14326, #14512, #8393, #8612, #8311 ),
 ( #13410, #2608, #13092, #2291, #7122, #7206, #1100, #14358, #3555, #12006, #6643, #2997, #7826, #4012, #1485, #6325, #366, #7589, #8763, #205, #7747, #5129, #442, #10107, #6404, #11367, #13795, #12616, #9958, #291, #1803, #11212, #14669, #14744, #3942, #11282, #8846, #2923, #11137, #525, #12459, #10182, #4165, #14899 ) ),
 .UNSPECIFIED., .T., .F., .F.,
 ( 4, 2, 4 ),
 ( 4, 2, 2, 2, 2, 2, 2, 2, 2, 2, 2, 2, 2, 2, 2, 2, 2, 2, 2, 2, 2, 4 ),
 ( 0.000000000000000000, 0.5000000000000000000, 1.000000000000000000 ),
 ( 0.000000000000000000, 0.01154246058414762008, 0.06319472280952896648, 0.1156547325041140800, 0.1678637871092111822, 0.2189476930995808979, 0.2714221776790743945, 0.3227197530690046334, 0.3747274728241424824, 0.4267432521036158555, 0.4780248536244998681, 0.5305055628088307662, 0.5815973485975094448, 0.6337991395759137170, 0.6855599279679012170, 0.7371634071600560167, 0.7894711232639126663, 0.8405207634104210346, 0.8929453349049019106, 0.9452650328228678900, 0.9965476795071586125, 1.000000000000000000 ),
 .UNSPECIFIED. ) ;
#4496=CARTESIAN_POINT ( 'NONE',  ( 209.6506722393607731, 33.81364540586627498, -6.382933553887647271 ) ) ;
#4522=DIRECTION ( 'NONE',  ( -0.7900120431063429871, 0.6130913241491365850, 0.000000000000000000 ) ) ;
#4526=CARTESIAN_POINT ( 'NONE',  ( 203.1202131991386182, 29.73909689272393564, -6.555651296533415717 ) ) ;
#4541=CARTESIAN_POINT ( 'NONE',  ( 207.1167095084715868, 46.15093117762712893, -7.185265714380067337 ) ) ;
#4546=LINE ( 'NONE', #3518, #736 ) ;
#4560=VECTOR ( 'NONE', #11119, 1000.000000000000227 ) ;
#4568=CARTESIAN_POINT ( 'NONE',  ( 0.000000000000000000, 0.000000000000000000, 0.000000000000000000 ) ) ;
#4585=ORIENTED_EDGE ( 'NONE', *, *, #1603, .F. ) ;
#4607=CARTESIAN_POINT ( 'NONE',  ( 191.4177849616493461, 42.04274826850978286, -7.631480755160323426 ) ) ;
#4617=CARTESIAN_POINT ( 'NONE',  ( 202.8882743124338504, 32.81631024066724933, -8.087096619718394663 ) ) ;
#4624=CARTESIAN_POINT ( 'NONE',  ( 201.8629198063431716, 32.54887535240757757, -8.146526315903498627 ) ) ;
#4654=CARTESIAN_POINT ( 'NONE',  ( 201.1886137893777970, 49.58779752487713210, -5.375724496774349603 ) ) ;
#4659=DIRECTION ( 'NONE',  ( -0.3662838836490099337, 0.9305003370641709015, 0.002288952263120960697 ) ) ;
#4665=EDGE_CURVE ( 'NONE', #10184, #9376, #1392, .T. ) ;
#4680=CARTESIAN_POINT ( 'NONE',  ( 211.8797403387081317, 42.53270508615055689, -3.012218501410035998 ) ) ;
#4693=CARTESIAN_POINT ( 'NONE',  ( 207.1325720688761294, 35.61275714886660637, -4.804596322733623914 ) ) ;
#4733=CARTESIAN_POINT ( 'NONE',  ( 208.7906731791537425, 42.14840350977979710, -9.001400940668622397 ) ) ;
#4762=CARTESIAN_POINT ( 'NONE',  ( 188.3692075015854357, 39.10978640110493387, -4.508345083535985509 ) ) ;
#4769=CIRCLE ( 'NONE', #9819, 1.499999999999992228 ) ;
#4774=CARTESIAN_POINT ( 'NONE',  ( 205.4319281802536068, 33.87189768065903905, -1.932853472788024440 ) ) ;
#4801=CARTESIAN_POINT ( 'NONE',  ( 162.8786896253216412, 17.13408854601560449, -5.884700754135287148 ) ) ;
#4809=CARTESIAN_POINT ( 'NONE',  ( 171.7208925888976978, 62.57671370024034729, -0.9107274384406883749 ) ) ;
#4820=CARTESIAN_POINT ( 'NONE',  ( 193.1767286061335653, 35.44822858574072910, -7.249992917093472933 ) ) ;
#4834=AXIS2_PLACEMENT_3D ( 'NONE', #5965, #15570, #1685 ) ;
#4849=CARTESIAN_POINT ( 'NONE',  ( 192.9079700310636269, 50.30505391962363149, -5.011923969639807019 ) ) ;
#4859=CARTESIAN_POINT ( 'NONE',  ( 191.4227524587821279, 39.61567282607229856, -2.929995994935606252 ) ) ;
#4889=FACE_OUTER_BOUND ( 'NONE', #6374, .T. ) ;
#4905=ORIENTED_EDGE ( 'NONE', *, *, #7414, .T. ) ;
#4910=CARTESIAN_POINT ( 'NONE',  ( 201.7654193689693045, 29.10045082804961325, -2.190250528083291570 ) ) ;
#4928=CARTESIAN_POINT ( 'NONE',  ( 207.2255354594468884, 50.38222520613008015, -5.636003230111601425 ) ) ;
#4935=CARTESIAN_POINT ( 'NONE',  ( 211.8917419932436985, 39.20340779279173660, -5.995121456379560954 ) ) ;
#4941=DIRECTION ( 'NONE',  ( 0.000000000000000000, 0.9569673715906177325, 0.2901955370279575286 ) ) ;
#4944=CARTESIAN_POINT ( 'NONE',  ( 201.3139613293953971, 49.56665511821758230, -6.809528532989353344 ) ) ;
#4948=CARTESIAN_POINT ( 'NONE',  ( 202.6027916890166694, 29.64969172180087398, -8.171549047034778468 ) ) ;
#4975=CARTESIAN_POINT ( 'NONE',  ( 193.0816233526163046, 46.15577860858359571, -4.879990690958216248 ) ) ;
#4983=CARTESIAN_POINT ( 'NONE',  ( 190.6253575848006960, 33.70309657413156401, -2.691919612340673673 ) ) ;
#5011=PRODUCT_DEFINITION_FORMATION_WITH_SPECIFIED_SOURCE ( 'ANY', '', #690, .NOT_KNOWN. ) ;
#5014=CARTESIAN_POINT ( 'NONE',  ( 203.2853005557455788, 48.75346994511389198, 0.6442813861133344089 ) ) ;
#5022=CARTESIAN_POINT ( 'NONE',  ( 203.0658429208174880, 48.83360436048501896, -0.9158339742359169477 ) ) ;
#5060=CARTESIAN_POINT ( 'NONE',  ( 192.8746960878046650, 31.41537247659151433, -2.569271051570655384 ) ) ;
#5080=CARTESIAN_POINT ( 'NONE',  ( 205.4339596421060889, 33.86846485884471747, -4.932823326473320336 ) ) ;
#5090=CARTESIAN_POINT ( 'NONE',  ( 201.2644297667355886, 32.15691159195442594, -0.6119088838163699862 ) ) ;
#5099=CARTESIAN_POINT ( 'NONE',  ( 201.7905037730716913, 32.52922036567187547, -6.577523224799477930 ) ) ;
#5129=CARTESIAN_POINT ( 'NONE',  ( 208.8051451104704768, 39.65587490144260840, -4.559632177755815086 ) ) ;
#5137=CARTESIAN_POINT ( 'NONE',  ( 204.1086650545086911, 51.64708631006858752, -0.9236185576248838736 ) ) ;
#5154=VERTEX_POINT ( 'NONE', #3642 ) ;
#5157=CARTESIAN_POINT ( 'NONE',  ( 205.4081958545874613, 47.87064854543508829, -4.057643371672452481 ) ) ;
#5162=ADVANCED_FACE ( 'NONE', ( #8545 ), #9888, .T. ) ;
#5165=CARTESIAN_POINT ( 'NONE',  ( 207.0901250877858217, 35.54806830018342367, -3.235595374952740855 ) ) ;
#5166=EDGE_LOOP ( 'NONE', ( #15387, #11778 ) ) ;
#5175=CARTESIAN_POINT ( 'NONE',  ( 194.8381067511959372, 47.88228248201940573, -3.436395123936771601 ) ) ;
#5214=CARTESIAN_POINT ( 'NONE',  ( 207.2900793066480674, 50.33932807692791300, -4.067002334276190290 ) ) ;
#5215=ORIENTED_EDGE ( 'NONE', *, *, #7718, .T. ) ;
#5231=CARTESIAN_POINT ( 'NONE',  ( 203.2140370934807834, 48.77700970988914264, -0.9247215889056725757 ) ) ;
#5245=ORIENTED_EDGE ( 'NONE', *, *, #6453, .F. ) ;
#5247=CARTESIAN_POINT ( 'NONE',  ( 191.3907470605235801, 42.09736693221333326, -1.487451979171016125 ) ) ;
#5257=VERTEX_POINT ( 'NONE', #9172 ) ;
#5313=CARTESIAN_POINT ( 'NONE',  ( 207.1164837741930569, 35.57719129110033407, -1.806778302941847159 ) ) ;
#5322=DIRECTION ( 'NONE',  ( 0.9296197478520976665, 0.3660421972118349521, -0.04266420354037676888 ) ) ;
#5328=CARTESIAN_POINT ( 'NONE',  ( 208.8002188652075972, 39.64064887424692785, -1.560527519332197022 ) ) ;
#5334=EDGE_CURVE ( 'NONE', #14252, #6288, #14183, .T. ) ;
#5373=VERTEX_POINT ( 'NONE', #5686 ) ;
#5395=CARTESIAN_POINT ( 'NONE',  ( 198.9111841706756536, 32.15857605477618364, -5.308824953579920347 ) ) ;
#5401=DIRECTION ( 'NONE',  ( 0.9296197478520976665, 0.3660421972118349521, -0.04266420354037676888 ) ) ;
#5412=CARTESIAN_POINT ( 'NONE',  ( 201.7406124912899941, 52.65652330452660834, -2.244206067705167396 ) ) ;
#5419=SHAPE_REPRESENTATION ( 'Recoil spring', ( #12337 ), #6298 ) ;
#5428=CARTESIAN_POINT ( 'NONE',  ( 170.2980342783642982, 56.44038842094546737, -0.9107274384406883749 ) ) ;
#5463=CARTESIAN_POINT ( 'NONE',  ( 211.8964099132376191, 42.41229301046570299, -5.872780407435223893 ) ) ;
#5477=CARTESIAN_POINT ( 'NONE',  ( 207.1167095084715868, 46.15093117762712893, -7.185265714380067337 ) ) ;
#5481=DIRECTION ( 'NONE',  ( 0.000000000000000000, 0.000000000000000000, -1.000000000000000000 ) ) ;
#5486=DIRECTION ( 'NONE',  ( -0.3662838836490099337, 0.9305003370641709015, 0.002288952263120960697 ) ) ;
#5491=CARTESIAN_POINT ( 'NONE',  ( 203.7958462291278749, 29.94547861640233322, -6.526400227122580944 ) ) ;
#5494=CARTESIAN_POINT ( 'NONE',  ( 202.1731860119849102, 31.08132011834958419, -8.150590381057213563 ) ) ;
#5517=VECTOR ( 'NONE', #12410, 1000.000000000000114 ) ;
#5536=CARTESIAN_POINT ( 'NONE',  ( 171.7208925888976978, 62.57671370024034729, -0.9107274384406883749 ) ) ;
#5541=CARTESIAN_POINT ( 'NONE',  ( 201.6516474359912934, 52.64960446646696113, -8.385050746608255778 ) ) ;
#5552=CARTESIAN_POINT ( 'NONE',  ( 201.2658342953964166, 49.58143373454755931, -3.806719548689701416 ) ) ;
#5567=ORIENTED_EDGE ( 'NONE', *, *, #3952, .F. ) ;
#5570=CARTESIAN_POINT ( 'NONE',  ( 209.6356879938037139, 47.96904352876332922, -5.622739983145865317 ) ) ;
#5592=STYLED_ITEM ( 'NONE', ( #1022 ), #642 ) ;
#5607=DIRECTION ( 'NONE',  ( -0.7900120431063429871, 0.6130913241491365850, 0.000000000000000000 ) ) ;
#5617=CARTESIAN_POINT ( 'NONE',  ( 209.6291075214908801, 33.76515323716659367, -3.385148507280513197 ) ) ;
#5627=CARTESIAN_POINT ( 'NONE',  ( 171.7208925888976978, 62.57671370024034729, -0.9107274384406881529 ) ) ;
#5643=CARTESIAN_POINT ( 'NONE',  ( 192.9601959511087728, 50.37386974367067438, -4.870874480120333416 ) ) ;
#5681=DIRECTION ( 'NONE',  ( 1.000000000000000000, 0.000000000000000000, 0.000000000000000000 ) ) ;
#5686=CARTESIAN_POINT ( 'NONE',  ( 203.8258924691278082, 51.74121150033466421, -0.9185252821640312870 ) ) ;
#5693=CARTESIAN_POINT ( 'NONE',  ( 211.8663679066739007, 39.14335912920272875, 0.001962313962203070510 ) ) ;
#5719=CARTESIAN_POINT ( 'NONE',  ( 209.6240687314160880, 33.75364762868482416, -9.385773361654676350 ) ) ;
#5729=CARTESIAN_POINT ( 'NONE',  ( 198.9393012728169765, 49.56711568108339350, -5.111368784863990378 ) ) ;
#5773=VERTEX_POINT ( 'NONE', #10484 ) ;
#5789=CIRCLE ( 'NONE', #219, 1.499999999999994227 ) ;
#5793=CARTESIAN_POINT ( 'NONE',  ( 191.3780708436489704, 41.94285887643944477, -4.625461852610818880 ) ) ;
#5806=CARTESIAN_POINT ( 'NONE',  ( 208.8060099514817978, 42.07246638764446089, -7.432400171711813996 ) ) ;
#5847=CARTESIAN_POINT ( 'NONE',  ( 211.8797403387081317, 42.53270508615055689, -3.012218501410035998 ) ) ;
#5851=ORIENTED_EDGE ( 'NONE', *, *, #2388, .F. ) ;
#5876=CARTESIAN_POINT ( 'NONE',  ( 198.9883150731717478, 32.15189384935130334, -6.877829860972676457 ) ) ;
#5885=CARTESIAN_POINT ( 'NONE',  ( 193.1007612367029367, 46.15997280778478995, -6.307360761128419036 ) ) ;
#5892=CARTESIAN_POINT ( 'NONE',  ( 207.1167095084715868, 46.15093117762712893, -7.185265714380067337 ) ) ;
#5921=CARTESIAN_POINT ( 'NONE',  ( 191.4177849616493461, 42.04274826850978286, -7.631480755160323426 ) ) ;
#5950=CARTESIAN_POINT ( 'NONE',  ( 192.9390872975532716, 31.37216231216662266, -4.138271986312449080 ) ) ;
#5963=CARTESIAN_POINT ( 'NONE',  ( 193.0950460371283839, 35.57958264137020876, -2.685405722344195389 ) ) ;
#5965=CARTESIAN_POINT ( 'NONE',  ( 152.8671246545933400, 7.480744990243093362, -7.157132912367466737 ) ) ;
#5972=CARTESIAN_POINT ( 'NONE',  ( 208.8124460758720033, 42.05191026284237665, -4.433604294307299298 ) ) ;
#6004=CARTESIAN_POINT ( 'NONE',  ( 205.3436520073863107, 47.91354567463725544, -5.626644267508417840 ) ) ;
#6014=AXIS2_PLACEMENT_3D ( 'NONE', #9187, #870, #790 ) ;
#6030=DIRECTION ( 'NONE',  ( -0.2258817899775119320, -0.9741547192086866813, 0.000000000000000000 ) ) ;
#6034=CARTESIAN_POINT ( 'NONE',  ( 202.4595012533446550, 32.68412682837883665, -9.685340726858029825 ) ) ;
#6040=AXIS2_PLACEMENT_3D ( 'NONE', #7453, #13190, #6030 ) ;
#6043=CIRCLE ( 'NONE', #4272, 1.499999999999988232 ) ;
#6044=CARTESIAN_POINT ( 'NONE',  ( 208.8002188652075972, 39.64064887424692785, -1.560527519332197022 ) ) ;
#6058=CARTESIAN_POINT ( 'NONE',  ( 202.8882743124338504, 32.81631024066724933, -8.087096619718394663 ) ) ;
#6088=ORIENTED_EDGE ( 'NONE', *, *, #7443, .T. ) ;
#6091=CARTESIAN_POINT ( 'NONE',  ( 193.1446408943811548, 35.52021409135998198, -4.254410606405073736 ) ) ;
#6097=CARTESIAN_POINT ( 'NONE',  ( 209.6025922774668118, 47.99519474844118605, -4.193309970723227309 ) ) ;
#6114=CARTESIAN_POINT ( 'NONE',  ( 209.6506722393607731, 33.81364540586627498, -6.382933553887647271 ) ) ;
#6123=CARTESIAN_POINT ( 'NONE',  ( 208.8276044750562335, 41.97590694738037342, -2.864603354092789100 ) ) ;
#6132=AXIS2_PLACEMENT_3D ( 'NONE', #10996, #7056, #3718 ) ;
#6143=PRODUCT_DEFINITION ( 'UNKNOWN', '', #5011, #9955 ) ;
#6149=CARTESIAN_POINT ( 'NONE',  ( 163.9288925978260067, 14.41035391906034491, -6.370175303308201364 ) ) ;
#6152=ORIENTED_EDGE ( 'NONE', *, *, #7718, .F. ) ;
#6163=EDGE_CURVE ( 'NONE', #8651, #5154, #4372, .T. ) ;
#6177=CARTESIAN_POINT ( 'NONE',  ( 209.5860849711743015, 48.02841048703755433, -7.191744956496605390 ) ) ;
#6195=CARTESIAN_POINT ( 'NONE',  ( 201.3139613293953971, 49.56665511821758230, -6.809528532989353344 ) ) ;
#6199=DIRECTION ( 'NONE',  ( 0.6130913241491352528, 0.7900120431063439863, -6.390853288715847897E-17 ) ) ;
#6204=CARTESIAN_POINT ( 'NONE',  ( 192.8103048780560584, 31.45858264101640600, -1.000270116828862133 ) ) ;
#6212=CARTESIAN_POINT ( 'NONE',  ( 207.0737247153217311, 35.51262227952910422, -0.2377773810599485560 ) ) ;
#6239=CARTESIAN_POINT ( 'NONE',  ( 208.8119396302737130, 39.73295740579614943, -6.128637076002331874 ) ) ;
#6249=CARTESIAN_POINT ( 'NONE',  ( 190.6680756494005209, 33.60499951150965359, -5.687464151445976945 ) ) ;
#6261=CYLINDRICAL_SURFACE ( 'NONE', #8721, 1.500000000000000444 ) ;
#6269=CARTESIAN_POINT ( 'NONE',  ( 208.8162124854775357, 42.04914431719598156, -1.433821094984975009 ) ) ;
#6279=CARTESIAN_POINT ( 'NONE',  ( 191.4070815280707052, 39.69144961696751039, -1.360995051912267106 ) ) ;
#6286=CARTESIAN_POINT ( 'NONE',  ( 194.8483215340629613, 47.90965193911861775, -4.864368187704507740 ) ) ;
#6288=VERTEX_POINT ( 'NONE', #654 ) ;
#6292=DIRECTION ( 'NONE',  ( -0.1562424607007877608, 0.2866315678550999668, -0.9452145987991775744 ) ) ;
#6298=( GEOMETRIC_REPRESENTATION_CONTEXT ( 3 ) GLOBAL_UNCERTAINTY_ASSIGNED_CONTEXT ( ( #2964 ) ) GLOBAL_UNIT_ASSIGNED_CONTEXT ( ( #13235, #7109, #14420 ) ) REPRESENTATION_CONTEXT ( 'NONE', 'WORKASPACE' ) );
#6325=CARTESIAN_POINT ( 'NONE',  ( 193.1265229109121435, 35.50728864820005981, -5.680987958736793075 ) ) ;
#6331=CARTESIAN_POINT ( 'NONE',  ( 211.8732981324650382, 39.22040580830856982, -1.567042559649178379 ) ) ;
#6354=CARTESIAN_POINT ( 'NONE',  ( 205.4699394944333051, 33.88363592193200446, -7.930995773285529182 ) ) ;
#6363=CARTESIAN_POINT ( 'NONE',  ( 211.8731694863154758, 39.16394563883312685, -2.997139605818726515 ) ) ;
#6372=CARTESIAN_POINT ( 'NONE',  ( 193.0950460371283839, 35.57958264137020876, -2.685405722344195389 ) ) ;
#6374=EDGE_LOOP ( 'NONE', ( #3046, #1676, #2884, #4585 ) ) ;
#6387=EDGE_LOOP ( 'NONE', ( #12046, #9559, #10907, #10179, #14683 ) ) ;
#6404=CARTESIAN_POINT ( 'NONE',  ( 205.4081958545874613, 47.87064854543508829, -4.057643371672452481 ) ) ;
#6419=AXIS2_PLACEMENT_3D ( 'NONE', #15591, #996, #12133 ) ;
#6449=CARTESIAN_POINT ( 'NONE',  ( 207.0901250877858217, 35.54806830018342367, -3.235595374952740855 ) ) ;
#6453=EDGE_CURVE ( 'NONE', #5257, #7692, #208, .T. ) ;
#6504=CARTESIAN_POINT ( 'NONE',  ( 172.0899380277727744, 70.88000906936352408, -0.9107274384406883749 ) ) ;
#6509=CARTESIAN_POINT ( 'NONE',  ( 193.1007612367029367, 46.15997280778478995, -6.307360761128419036 ) ) ;
#6528=CARTESIAN_POINT ( 'NONE',  ( 198.8340532681795594, 32.16525826020106393, -3.739820046187162905 ) ) ;
#6576=CIRCLE ( 'NONE', #15363, 1.499999999999995115 ) ;
#6606=CARTESIAN_POINT ( 'NONE',  ( 207.2819921120892275, 50.35227183911742088, -8.638656677529437999 ) ) ;
#6643=CARTESIAN_POINT ( 'NONE',  ( 198.8634854004546071, 49.55149448133588663, -6.680369717582868461 ) ) ;
#6647=ORIENTED_EDGE ( 'NONE', *, *, #3952, .T. ) ;
#6672=CARTESIAN_POINT ( 'NONE',  ( 193.1007612367029367, 46.15997280778478995, -6.307360761128419036 ) ) ;
#6688=CARTESIAN_POINT ( 'NONE',  ( 211.9100270530500154, 42.38063601863193242, 0.1257832527464326222 ) ) ;
#6732=CARTESIAN_POINT ( 'NONE',  ( 209.5364819485449175, 48.08777744531177945, -8.760749929847346351 ) ) ;
#6744=CARTESIAN_POINT ( 'NONE',  ( 194.7691866843436799, 33.87697957786221536, -2.559886773443665220 ) ) ;
#6757=CARTESIAN_POINT ( 'NONE',  ( 188.3378656401271201, 39.26133998289535043, -1.370343197488200548 ) ) ;
#6764=AXIS2_PLACEMENT_3D ( 'NONE', #8219, #6869, #10722 ) ;
#6770=DIRECTION ( 'NONE',  ( -0.7900120431063429871, 0.6130913241491365850, 0.000000000000000000 ) ) ;
#6793=ORIENTED_EDGE ( 'NONE', *, *, #15180, .F. ) ;
#6798=CARTESIAN_POINT ( 'NONE',  ( 166.7445055987502656, 66.43865443379108626, -0.9107274384406879308 ) ) ;
#6804=AXIS2_PLACEMENT_3D ( 'NONE', #566, #12723, #7865 ) ;
#6807=CARTESIAN_POINT ( 'NONE',  ( 198.5455061167297117, 29.08454594588317477, -3.885748181069116569 ) ) ;
#6812=EDGE_LOOP ( 'NONE', ( #10342, #5215, #10858, #11371 ) ) ;
#6818=CARTESIAN_POINT ( 'NONE',  ( 207.1288103955774318, 46.12660085639766550, -4.186765234109192768 ) ) ;
#6837=CARTESIAN_POINT ( 'NONE',  ( 201.6895650671498288, 29.08490409614774208, -0.6212496039192949571 ) ) ;
#6865=CARTESIAN_POINT ( 'NONE',  ( 203.4093511297053851, 50.30250970312692971, -0.9107274384406970347 ) ) ;
#6869=DIRECTION ( 'NONE',  ( 0.000000000000000000, 0.000000000000000000, -1.000000000000000000 ) ) ;
#6883=DIRECTION ( 'NONE',  ( 0.000000000000000000, 0.000000000000000000, -1.000000000000000000 ) ) ;
#6888=CARTESIAN_POINT ( 'NONE',  ( 207.4341467637200651, 31.47497422714618764, -9.505705820141434614 ) ) ;
#6914=CARTESIAN_POINT ( 'NONE',  ( 211.8731694863154758, 39.16394563883312685, -2.997139605818726515 ) ) ;
#6964=CARTESIAN_POINT ( 'NONE',  ( 207.3850704934720284, 31.45434786795649984, -6.508326106789642296 ) ) ;
#6970=DIRECTION ( 'NONE',  ( 0.9296197478520976665, 0.3660421972118349521, -0.04266420354037676888 ) ) ;
#6992=CARTESIAN_POINT ( 'NONE',  ( 201.3303440367248243, 32.15585396293944598, -6.755036635249508592 ) ) ;
#6999=CARTESIAN_POINT ( 'NONE',  ( 193.1265229109121435, 35.50728864820005981, -5.680987958736793075 ) ) ;
#7038=ADVANCED_FACE ( 'NONE', ( #11030 ), #8845, .T. ) ;
#7056=DIRECTION ( 'NONE',  ( 0.9296197478520976665, 0.3660421972118349521, -0.04266420354037676888 ) ) ;
#7059=AXIS2_PLACEMENT_3D ( 'NONE', #6504, #11304, #14923 ) ;
#7070=CARTESIAN_POINT ( 'NONE',  ( 207.3736904795575811, 50.31851200600168994, -2.642755332960478043 ) ) ;
#7082=CARTESIAN_POINT ( 'NONE',  ( 207.1663125311009992, 46.09156421935289671, -5.616260741029326375 ) ) ;
#7108=EDGE_CURVE ( 'NONE', #11153, #14187, #2277, .T. ) ;
#7109=( NAMED_UNIT ( * ) PLANE_ANGLE_UNIT ( ) SI_UNIT ( $, .RADIAN. ) );
#7122=CARTESIAN_POINT ( 'NONE',  ( 207.1131222881253393, 35.56952893079440514, -7.807171136772324438 ) ) ;
#7150=CARTESIAN_POINT ( 'NONE',  ( 193.0579178353149246, 46.09544038230585272, -7.876361695281355324 ) ) ;
#7163=CARTESIAN_POINT ( 'NONE',  ( 194.7957337413261030, 33.86335648926068842, -5.558215102112974648 ) ) ;
#7206=CARTESIAN_POINT ( 'NONE',  ( 208.8186272397570349, 39.68461847005694665, -7.558035125831273682 ) ) ;
#7232=CARTESIAN_POINT ( 'NONE',  ( 211.8867585259220050, 39.31811064754020890, -6.135149402309513000 ) ) ;
#7237=AXIS2_PLACEMENT_3D ( 'NONE', #12274, #6292, #9855 ) ;
#7240=CARTESIAN_POINT ( 'NONE',  ( 208.8162124854775357, 42.04914431719598156, -1.433821094984975009 ) ) ;
#7279=CARTESIAN_POINT ( 'NONE',  ( 201.9353358396146234, 32.56853033914327966, -9.715529407007519325 ) ) ;
#7280=SURFACE_SIDE_STYLE ('',( #10746 ) ) ;
#7304=CARTESIAN_POINT ( 'NONE',  ( 207.1592428330643827, 35.64176030267155681, -3.375779224823745928 ) ) ;
#7316=CARTESIAN_POINT ( 'NONE',  ( 211.9048830940805885, 42.38452776791458376, -2.873977808594950112 ) ) ;
#7350=DIRECTION ( 'NONE',  ( 0.000000000000000000, 0.000000000000000000, -1.000000000000000000 ) ) ;
#7365=CARTESIAN_POINT ( 'NONE',  ( 211.8948836958790594, 42.45667055239124466, -1.443217624331801563 ) ) ;
#7386=CARTESIAN_POINT ( 'NONE',  ( 193.0950460371283839, 35.57958264137020876, -2.685405722344195389 ) ) ;
#7396=CARTESIAN_POINT ( 'NONE',  ( 188.3076603040395582, 42.49356297222218615, -1.493920802967548367 ) ) ;
#7414=EDGE_CURVE ( 'NONE', #6288, #14252, #982, .T. ) ;
#7433=CARTESIAN_POINT ( 'NONE',  ( 198.7876695280922661, 49.53587328158837977, -8.249370650301745655 ) ) ;
#7443=EDGE_CURVE ( 'NONE', #5773, #11153, #2774, .T. ) ;
#7453=CARTESIAN_POINT ( 'NONE',  ( 203.4093511297050725, 50.30250970312702208, -0.9107274384406883749 ) ) ;
#7457=CARTESIAN_POINT ( 'NONE',  ( 205.4319281802536068, 33.87189768065903905, -1.932853472788024440 ) ) ;
#7466=CARTESIAN_POINT ( 'NONE',  ( 207.1782284445936284, 46.06712597851176838, -2.617760425820522041 ) ) ;
#7474=CARTESIAN_POINT ( 'NONE',  ( 207.1164837741930569, 35.57719129110033407, -1.806778302941847159 ) ) ;
#7476=ORIENTED_EDGE ( 'NONE', *, *, #8722, .F. ) ;
#7490=CARTESIAN_POINT ( 'NONE',  ( 166.9217645774054120, 62.57671370024034729, -0.9107274384406883749 ) ) ;
#7504=ORIENTED_EDGE ( 'NONE', *, *, #7414, .F. ) ;
#7528=EDGE_CURVE ( 'NONE', #8873, #9626, #10591, .T. ) ;
#7534=CARTESIAN_POINT ( 'NONE',  ( 194.7957337413261030, 33.86335648926068842, -5.558215102112974648 ) ) ;
#7545=CARTESIAN_POINT ( 'NONE',  ( 209.6356879938037139, 47.96904352876332922, -5.622739983145865317 ) ) ;
#7553=CARTESIAN_POINT ( 'NONE',  ( 201.3910773252651438, 49.55986643532389735, -5.240523689774838623 ) ) ;
#7589=CARTESIAN_POINT ( 'NONE',  ( 198.9111841706756536, 32.15857605477618364, -5.308824953579920347 ) ) ;
#7595=CARTESIAN_POINT ( 'NONE',  ( 203.8258924691278082, 51.74121150033466421, -0.9185252821640312870 ) ) ;
#7617=CARTESIAN_POINT ( 'NONE',  ( 169.1145417280692698, 64.59938046134368506, -0.9107274384406877088 ) ) ;
#7635=CARTESIAN_POINT ( 'NONE',  ( 201.1780093772972009, 32.12620995903681376, -3.617034841014101776 ) ) ;
#7663=ORIENTED_EDGE ( 'NONE', *, *, #7108, .T. ) ;
#7675=CARTESIAN_POINT ( 'NONE',  ( 211.8799640061187404, 39.24102814318666788, -4.566144504064119758 ) ) ;
#7685=ORIENTED_EDGE ( 'NONE', *, *, #1097, .T. ) ;
#7692=VERTEX_POINT ( 'NONE', #12417 ) ;
#7694=CARTESIAN_POINT ( 'NONE',  ( 201.8629198063431716, 32.54887535240757757, -8.146526315903498627 ) ) ;
#7715=CARTESIAN_POINT ( 'NONE',  ( 207.1782284445936284, 46.06712597851176838, -2.617760425820522041 ) ) ;
#7718=EDGE_CURVE ( 'NONE', #7692, #6288, #13860, .T. ) ;
#7747=CARTESIAN_POINT ( 'NONE',  ( 207.1325720688761294, 35.61275714886660637, -4.804596322733623914 ) ) ;
#7771=CARTESIAN_POINT ( 'NONE',  ( 205.4081958545874613, 47.87064854543508829, -4.057643371672452481 ) ) ;
#7791=CARTESIAN_POINT ( 'NONE',  ( 198.3913412372077687, 29.09831693401786268, -0.7477385443502184703 ) ) ;
#7798=AXIS2_PLACEMENT_3D ( 'NONE', #1371, #2489, #4941 ) ;
#7826=CARTESIAN_POINT ( 'NONE',  ( 193.1007612367029367, 46.15997280778478995, -6.307360761128419036 ) ) ;
#7846=CARTESIAN_POINT ( 'NONE',  ( 193.0454511798755846, 35.63895119138042133, -1.116400838283317043 ) ) ;
#7858=CARTESIAN_POINT ( 'NONE',  ( 191.3844089520862894, 42.02011290432638901, -3.056456915890917170 ) ) ;
#7865=DIRECTION ( 'NONE',  ( -0.3662838836490107108, 0.9305003370641705684, 0.002288952263120965468 ) ) ;
#7874=CARTESIAN_POINT ( 'NONE',  ( 203.2625657313046190, 29.78760669494945645, -9.693656633365744568 ) ) ;
#7899=EDGE_CURVE ( 'NONE', #10985, #14187, #8905, .T. ) ;
#7922=CARTESIAN_POINT ( 'NONE',  ( 211.9100270530500154, 42.38063601863193242, 0.1257832527464326222 ) ) ;
#7933=CARTESIAN_POINT ( 'NONE',  ( 207.1325720688761294, 35.61275714886660637, -4.804596322733623914 ) ) ;
#7942=CARTESIAN_POINT ( 'NONE',  ( 163.3793289068652257, 15.80605437029538507, -6.370175303308196924 ) ) ;
#7949=CARTESIAN_POINT ( 'NONE',  ( 207.4107378919655673, 50.26574450011962369, -5.500654858001599479 ) ) ;
#7961=CARTESIAN_POINT ( 'NONE',  ( 172.0899380277727744, 70.88000906936352408, -0.9107274384406883749 ) ) ;
#7964=CIRCLE ( 'NONE', #2909, 1.500000000000000666 ) ;
#7977=VECTOR ( 'NONE', #9053, 1000.000000000000227 ) ;
#7997=CARTESIAN_POINT ( 'NONE',  ( 192.9390872975532716, 31.37216231216662266, -4.138271986312449080 ) ) ;
#8019=DIRECTION ( 'NONE',  ( -0.3297523322010256219, -0.9440639390088612082, 0.002584273796984222320 ) ) ;
#8022=UNCERTAINTY_MEASURE_WITH_UNIT (LENGTH_MEASURE( 1.000000000000000082E-05 ), #12007, 'distance_accuracy_value', 'NONE');
#8023=CARTESIAN_POINT ( 'NONE',  ( 201.7245916543302826, 29.07256658421868423, -6.764440628860102223 ) ) ;
#8028=VECTOR ( 'NONE', #281, 999.9999999999998863 ) ;
#8080=CARTESIAN_POINT ( 'NONE',  ( 209.5435894037482285, 33.63601521402413397, -0.2471466635189603911 ) ) ;
#8102=VECTOR ( 'NONE', #15373, 1000.000000000000114 ) ;
#8111=CARTESIAN_POINT ( 'NONE',  ( 201.5722569949026877, 29.04292258031605556, -3.626438834624695406 ) ) ;
#8126=TOROIDAL_SURFACE ( 'NONE', #8385, 4.799128011492294732, 1.499999999999997113 ) ;
#8146=ORIENTED_EDGE ( 'NONE', *, *, #9692, .T. ) ;
#8147=DIRECTION ( 'NONE',  ( 0.000000000000000000, 0.000000000000000000, 1.000000000000000000 ) ) ;
#8156=CIRCLE ( 'NONE', #13165, 3.299128011492291623 ) ;
#8160=CARTESIAN_POINT ( 'NONE',  ( 188.3266922173125124, 39.20571348140700252, -7.512715813640810758 ) ) ;
#8187=CARTESIAN_POINT ( 'NONE',  ( 205.3852585099181454, 47.89158942159311039, -8.629264428576009394 ) ) ;
#8191=ADVANCED_FACE ( 'NONE', ( #693 ), #56, .T. ) ;
#8200=CARTESIAN_POINT ( 'NONE',  ( 191.4322133549729585, 42.19665789901188901, -4.493471110936619439 ) ) ;
#8219=CARTESIAN_POINT ( 'NONE',  ( 171.7208925888976978, 62.57671370024034729, -0.9107274384406883749 ) ) ;
#8248=CARTESIAN_POINT ( 'NONE',  ( 171.7208925888976978, 62.57671370024034729, -0.9107274384406883749 ) ) ;
#8260=CARTESIAN_POINT ( 'NONE',  ( 207.1750190499664370, 35.67744599754978907, -6.373597270514506974 ) ) ;
#8270=CARTESIAN_POINT ( 'NONE',  ( 193.1249951165660548, 46.22013307728793308, -3.310989833511668756 ) ) ;
#8277=DIRECTION ( 'NONE',  ( 0.5602235199536453880, 0.8138631617988981715, 0.1541958545404129299 ) ) ;
#8278=CARTESIAN_POINT ( 'NONE',  ( 208.8186272397570349, 39.68461847005694665, -7.558035125831273682 ) ) ;
#8281=CARTESIAN_POINT ( 'NONE',  ( 202.8882743124338504, 32.81631024066724933, -8.087096619718394663 ) ) ;
#8311=CARTESIAN_POINT ( 'NONE',  ( 202.8426534586648700, 48.90729187601812811, -2.475854291071949209 ) ) ;
#8312=SURFACE_STYLE_USAGE ( .BOTH. , #7280 ) ;
#8336=CARTESIAN_POINT ( 'NONE',  ( 207.0671064858421744, 46.21029813590134694, -8.754270687730807410 ) ) ;
#8349=CARTESIAN_POINT ( 'NONE',  ( 207.1131222881253393, 35.56952893079440514, -7.807171136772324438 ) ) ;
#8355=DIRECTION ( 'NONE',  ( -0.9741547192086869034, 0.2258817899775114879, 0.000000000000000000 ) ) ;
#8385=AXIS2_PLACEMENT_3D ( 'NONE', #4809, #2041, #14270 ) ;
#8393=CARTESIAN_POINT ( 'NONE',  ( 203.1427736312160164, 48.80054947466439330, -2.493724563924679671 ) ) ;
#8418=CARTESIAN_POINT ( 'NONE',  ( 208.8119396302737130, 39.73295740579614943, -6.128637076002331874 ) ) ;
#8420=DIRECTION ( 'NONE',  ( 0.000000000000000000, 0.000000000000000000, -1.000000000000000000 ) ) ;
#8422=CARTESIAN_POINT ( 'NONE',  ( 152.8671246545933400, 7.480744990243093362, -7.157132912367466737 ) ) ;
#8428=CARTESIAN_POINT ( 'NONE',  ( 205.4496313998743915, 47.84832575209421890, -7.060263518810960370 ) ) ;
#8437=CARTESIAN_POINT ( 'NONE',  ( 191.4249991583111523, 42.11970308376083949, -6.062475933048471433 ) ) ;
#8465=CARTESIAN_POINT ( 'NONE',  ( 193.0579178353149246, 46.09544038230585272, -7.876361695281355324 ) ) ;
#8492=CARTESIAN_POINT ( 'NONE',  ( 201.4161383703745400, 32.18800505576257365, -3.749910732146560122 ) ) ;
#8500=CARTESIAN_POINT ( 'NONE',  ( 205.4081958545874613, 47.87064854543508829, -4.057643371672452481 ) ) ;
#8517=CARTESIAN_POINT ( 'NONE',  ( 170.6368569633305583, 57.90162049975850067, -0.9107274384406883749 ) ) ;
#8536=CARTESIAN_POINT ( 'NONE',  ( 208.7972876766878016, 42.12791357830437988, -6.002605234521809052 ) ) ;
#8542=CARTESIAN_POINT ( 'NONE',  ( 207.3749241153878700, 31.42506699505091916, -7.936699686978753832 ) ) ;
#8545=FACE_OUTER_BOUND ( 'NONE', #15546, .T. ) ;
#8561=CARTESIAN_POINT ( 'NONE',  ( 208.8060099514817978, 42.07246638764446089, -7.432400171711813996 ) ) ;
#8569=AXIS2_PLACEMENT_3D ( 'NONE', #10861, #6199, #11012 ) ;
#8574=CARTESIAN_POINT ( 'NONE',  ( 194.7312355367470786, 33.90632498363353164, -3.989214208820068386 ) ) ;
#8584=CARTESIAN_POINT ( 'NONE',  ( 194.7891036845171300, 47.85977741052224133, -6.433373108600371815 ) ) ;
#8603=CARTESIAN_POINT ( 'NONE',  ( 203.4093511297050725, 50.30250970312702208, -0.9107274384406883749 ) ) ;
#8612=CARTESIAN_POINT ( 'NONE',  ( 202.9941614129404286, 48.85583040772959862, -2.484837107663659506 ) ) ;
#8619=CARTESIAN_POINT ( 'NONE',  ( 188.3013221956022392, 42.41630894433524190, -3.062925739686887638 ) ) ;
#8633=CARTESIAN_POINT ( 'NONE',  ( 163.3793289068652541, 15.80605437029534954, -6.370175303308202253 ) ) ;
#8635=FACE_OUTER_BOUND ( 'NONE', #13922, .T. ) ;
#8639=CARTESIAN_POINT ( 'NONE',  ( 194.7891036845171300, 47.85977741052224133, -6.433373108600371815 ) ) ;
#8650=CARTESIAN_POINT ( 'NONE',  ( 208.7983505906672121, 39.57879239708907448, -2.990627279509298742 ) ) ;
#8651=VERTEX_POINT ( 'NONE', #4948 ) ;
#8661=CARTESIAN_POINT ( 'NONE',  ( 201.2658342953964166, 49.58143373454755931, -3.806719548689701416 ) ) ;
#8699=CARTESIAN_POINT ( 'NONE',  ( 201.6484243246164851, 29.05774458226736812, -5.195439731742398592 ) ) ;
#8717=CARTESIAN_POINT ( 'NONE',  ( 202.8882743124338504, 32.81631024066724933, -8.087096619718394663 ) ) ;
#8721=AXIS2_PLACEMENT_3D ( 'NONE', #8633, #231, #14689 ) ;
#8722=EDGE_CURVE ( 'NONE', #5154, #10184, #13291, .T. ) ;
#8725=CARTESIAN_POINT ( 'NONE',  ( 207.2666510146856069, 31.35441966018789728, -3.370316356820458381 ) ) ;
#8733=CARTESIAN_POINT ( 'NONE',  ( 194.7691866843436799, 33.87697957786221536, -2.559886773443665220 ) ) ;
#8763=CARTESIAN_POINT ( 'NONE',  ( 201.2541767070109984, 32.14103196098812987, -5.186035738131804962 ) ) ;
#8791=CARTESIAN_POINT ( 'NONE',  ( 202.9941614129404286, 48.85583040772959862, -2.484837107663659506 ) ) ;
#8810=CARTESIAN_POINT ( 'NONE',  ( 194.7312355367470786, 33.90632498363353164, -3.989214208820068386 ) ) ;
#8845=TOROIDAL_SURFACE ( 'NONE', #10352, 21.91351791792154202, 1.499999999999997113 ) ;
#8846=CARTESIAN_POINT ( 'NONE',  ( 207.1164837741930569, 35.57719129110033407, -1.806778302941847159 ) ) ;
#8855=CARTESIAN_POINT ( 'NONE',  ( 211.8810731409095922, 42.48823013260103920, -7.441781176392031405 ) ) ;
#8872=PLANE ( 'NONE',  #7059 ) ;
#8873=VERTEX_POINT ( 'NONE', #6149 ) ;
#8876=CARTESIAN_POINT ( 'NONE',  ( 205.4526553411199359, 47.86694802938139759, -2.633259993550844502 ) ) ;
#8878=CARTESIAN_POINT ( 'NONE',  ( 207.1131222881253393, 35.56952893079440514, -7.807171136772324438 ) ) ;
#8897=CARTESIAN_POINT ( 'NONE',  ( 203.2140370934807834, 48.77700970988914264, -0.9247215889056725757 ) ) ;
#8905=CIRCLE ( 'NONE', #6132, 1.500000000000000666 ) ;
#8958=CARTESIAN_POINT ( 'NONE',  ( 208.8186272397570349, 39.68461847005694665, -7.558035125831273682 ) ) ;
#8974=CARTESIAN_POINT ( 'NONE',  ( 191.4070815280707052, 39.69144961696751039, -1.360995051912267106 ) ) ;
#9020=CARTESIAN_POINT ( 'NONE',  ( 202.4110361843541455, 29.59410989755560806, -6.585651355106874050 ) ) ;
#9031=CARTESIAN_POINT ( 'NONE',  ( 201.2541767070109984, 32.14103196098812987, -5.186035738131804962 ) ) ;
#9032=CARTESIAN_POINT ( 'NONE',  ( 170.6368569633305583, 57.90162049975850067, -0.9107274384406883749 ) ) ;
#9044=ORIENTED_EDGE ( 'NONE', *, *, #12063, .T. ) ;
#9046=CARTESIAN_POINT ( 'NONE',  ( 209.5385712735872517, 33.62447922832576097, -6.247773722084159154 ) ) ;
#9047=ORIENTED_EDGE ( 'NONE', *, *, #7528, .T. ) ;
#9053=DIRECTION ( 'NONE',  ( 0.9296197478520974444, 0.3660421972118351741, -0.04266420354037655377 ) ) ;
#9061=CIRCLE ( 'NONE', #15087, 1.499999999999994227 ) ;
#9101=CARTESIAN_POINT ( 'NONE',  ( 198.3593989614203963, 52.60648038231462920, -8.258707374242266752 ) ) ;
#9113=CARTESIAN_POINT ( 'NONE',  ( 203.0658429208174880, 48.83360436048501896, -0.9158339742359169477 ) ) ;
#9129=CARTESIAN_POINT ( 'NONE',  ( 211.8917419932436985, 39.20340779279173660, -5.995121456379560954 ) ) ;
#9157=DIRECTION ( 'NONE',  ( -0.3297523322010256219, -0.9440639390088612082, 0.002584273796984222320 ) ) ;
#9172=CARTESIAN_POINT ( 'NONE',  ( 168.4217645774054120, 62.57671370024034729, -0.9107274384406881529 ) ) ;
#9180=CARTESIAN_POINT ( 'NONE',  ( 192.8417602520171670, 50.27412068648693122, -8.008884321912063342 ) ) ;
#9185=EDGE_LOOP ( 'NONE', ( #3236, #6647, #12499, #4229 ) ) ;
#9187=CARTESIAN_POINT ( 'NONE',  ( 171.7208925888976978, 62.57671370024034729, -0.9107274384406883749 ) ) ;
#9188=ORIENTED_EDGE ( 'NONE', *, *, #9984, .F. ) ;
#9189=CARTESIAN_POINT ( 'NONE',  ( 194.7957337413261030, 33.86335648926068842, -5.558215102112974648 ) ) ;
#9205=CARTESIAN_POINT ( 'NONE',  ( 192.8417602520171670, 50.27412068648693122, -8.008884321912063342 ) ) ;
#9207=DIRECTION ( 'NONE',  ( 0.9296197478520975555, 0.3660421972118350631, -0.04266420354037653295 ) ) ;
#9254=CARTESIAN_POINT ( 'NONE',  ( 204.1803465669382547, 51.62486026858844212, 0.6453845751958426913 ) ) ;
#9279=CARTESIAN_POINT ( 'NONE',  ( 203.9760488007458719, 51.69772753023573131, 0.6543994141905550288 ) ) ;
#9286=TOROIDAL_SURFACE ( 'NONE', #6764, 4.799128011492294732, 1.499999999999997113 ) ;
#9312=EDGE_CURVE ( 'NONE', #7692, #5257, #3805, .T. ) ;
#9330=CARTESIAN_POINT ( 'NONE',  ( 211.8745662956760896, 42.53653439883859022, -6.011979689023970508 ) ) ;
#9333=FILL_AREA_STYLE ('',( #10830 ) ) ;
#9356=CARTESIAN_POINT ( 'NONE',  ( 209.5364819485449175, 48.08777744531177945, -8.760749929847346351 ) ) ;
#9376=VERTEX_POINT ( 'NONE', #5428 ) ;
#9402=CARTESIAN_POINT ( 'NONE',  ( 211.9051874564029561, 39.35763625820981559, -9.133132850359100274 ) ) ;
#9430=CARTESIAN_POINT ( 'NONE',  ( 191.4069380837317453, 39.61051162384328705, -7.503330758807070566 ) ) ;
#9445=CARTESIAN_POINT ( 'NONE',  ( 208.8186272397570349, 39.68461847005694665, -7.558035125831273682 ) ) ;
#9474=DIRECTION ( 'NONE',  ( -0.7900120431063429871, 0.6130913241491365850, 0.000000000000000000 ) ) ;
#9481=CARTESIAN_POINT ( 'NONE',  ( 205.3852585099181454, 47.89158942159311039, -8.629264428576009394 ) ) ;
#9483=( NAMED_UNIT ( * ) SI_UNIT ( $, .STERADIAN. ) SOLID_ANGLE_UNIT ( ) );
#9508=CARTESIAN_POINT ( 'NONE',  ( 207.0793923465612352, 46.18607573428356972, -5.755770042397863051 ) ) ;
#9515=CARTESIAN_POINT ( 'NONE',  ( 208.8124460758720033, 42.05191026284237665, -4.433604294307299298 ) ) ;
#9558=CARTESIAN_POINT ( 'NONE',  ( 198.8104769829885754, 49.54338459298288200, -5.250705761417654216 ) ) ;
#9559=ORIENTED_EDGE ( 'NONE', *, *, #1415, .T. ) ;
#9573=CIRCLE ( 'NONE', #6804, 1.499999999999997558 ) ;
#9575=EDGE_LOOP ( 'NONE', ( #11609, #11453, #7685, #3653, #12640 ) ) ;
#9585=CARTESIAN_POINT ( 'NONE',  ( 190.6749524420355328, 33.64372802412135144, -4.260924496400990691 ) ) ;
#9599=CARTESIAN_POINT ( 'NONE',  ( 203.0658429208174880, 48.83360436048501896, -0.9158339742359169477 ) ) ;
#9618=ADVANCED_FACE ( 'NONE', ( #3602 ), #14934, .T. ) ;
#9620=DIRECTION ( 'NONE',  ( -0.9741547192086867923, 0.2258817899775115157, 1.688901894271609290E-28 ) ) ;
#9626=VERTEX_POINT ( 'NONE', #9904 ) ;
#9630=CARTESIAN_POINT ( 'NONE',  ( 171.7208925888976978, 62.57671370024034729, -0.9107274384406881529 ) ) ;
#9641=CARTESIAN_POINT ( 'NONE',  ( 207.0671064858421744, 46.21029813590134694, -8.754270687730807410 ) ) ;
#9667=CARTESIAN_POINT ( 'NONE',  ( 198.9643688939780191, 32.15902683440354082, -3.879216492611309519 ) ) ;
#9677=CARTESIAN_POINT ( 'NONE',  ( 194.7691866843436799, 33.87697957786221536, -2.559886773443665220 ) ) ;
#9692=EDGE_CURVE ( 'NONE', #5257, #14252, #2552, .T. ) ;
#9745=CARTESIAN_POINT ( 'NONE',  ( 204.0369835420791276, 51.66931235154874003, -2.492621690445610216 ) ) ;
#9755=CARTESIAN_POINT ( 'NONE',  ( 198.5423134874356208, 52.64753739496011065, -2.122073255223759780 ) ) ;
#9769=FACE_OUTER_BOUND ( 'NONE', #6387, .T. ) ;
#9799=CARTESIAN_POINT ( 'NONE',  ( 209.5898355175288543, 48.01761212650198729, -1.192236766262033232 ) ) ;
#9819=AXIS2_PLACEMENT_3D ( 'NONE', #13998, #3189, #8019 ) ;
#9825=CARTESIAN_POINT ( 'NONE',  ( 201.2658342953964166, 49.58143373454755931, -3.806719548689701416 ) ) ;
#9830=DIRECTION ( 'NONE',  ( -0.8204839007831782327, 0.5707893219124419160, -0.03171306586179808984 ) ) ;
#9837=CARTESIAN_POINT ( 'NONE',  ( 209.5657782771801578, 33.68426770849990959, -3.244931658323684687 ) ) ;
#9849=CARTESIAN_POINT ( 'NONE',  ( 205.5810540386909508, 47.77928077683765906, 0.5047415929677595559 ) ) ;
#9855=DIRECTION ( 'NONE',  ( 0.000000000000000000, 0.9569673715906176215, 0.2901955370279575286 ) ) ;
#9885=CARTESIAN_POINT ( 'NONE',  ( 198.4352148337827657, 52.62210158206652721, -6.689706441523388669 ) ) ;
#9888=CYLINDRICAL_SURFACE ( 'NONE', #3358, 1.499999999999994227 ) ;
#9904=CARTESIAN_POINT ( 'NONE',  ( 163.8799681884088955, 14.47802019457520473, -6.855649852481113804 ) ) ;
#9913=CARTESIAN_POINT ( 'NONE',  ( 201.3430548014149792, 49.57506994421799362, -2.237714600605053228 ) ) ;
#9923=CARTESIAN_POINT ( 'NONE',  ( 191.3844089520862894, 42.02011290432638901, -3.056456915890917170 ) ) ;
#9955=PRODUCT_DEFINITION_CONTEXT ( 'detailed design', #15611, 'design' ) ;
#9958=CARTESIAN_POINT ( 'NONE',  ( 193.1249951165660548, 46.22013307728793308, -3.310989833511668756 ) ) ;
#9984=EDGE_CURVE ( 'NONE', #8651, #5373, #15542, .T. ) ;
#9985=CARTESIAN_POINT ( 'NONE',  ( 208.8186272397570349, 39.68461847005694665, -7.558035125831273682 ) ) ;
#9994=CARTESIAN_POINT ( 'NONE',  ( 205.3727474927790411, 33.82195144205066839, -0.3638485434072702973 ) ) ;
#10002=CARTESIAN_POINT ( 'NONE',  ( 201.3402840685550643, 32.17245832385849980, -2.180909807981465054 ) ) ;
#10056=CARTESIAN_POINT ( 'NONE',  ( 203.2140370934807834, 48.77700970988914264, -0.9247215889056725757 ) ) ;
#10061=CARTESIAN_POINT ( 'NONE',  ( 163.3793289068652257, 15.80605437029538507, -6.370175303308196924 ) ) ;
#10065=ORIENTED_EDGE ( 'NONE', *, *, #5334, .T. ) ;
#10072=CARTESIAN_POINT ( 'NONE',  ( 205.5168546899054434, 47.82311440310952833, -1.064259200291542529 ) ) ;
#10073=ORIENTED_EDGE ( 'NONE', *, *, #7443, .F. ) ;
#10078=DIRECTION ( 'NONE',  ( -0.1562424607007877608, 0.2866315678550999668, -0.9452145987991775744 ) ) ;
#10107=CARTESIAN_POINT ( 'NONE',  ( 207.1288103955774318, 46.12660085639766550, -4.186765234109192768 ) ) ;
#10153=CARTESIAN_POINT ( 'NONE',  ( 202.3171501287270644, 32.63561614260228794, -6.547335233887139339 ) ) ;
#10157=CARTESIAN_POINT ( 'NONE',  ( 170.6931741512129577, -3.595212766542494887, -13.46247879130521952 ) ) ;
#10161=ORIENTED_EDGE ( 'NONE', *, *, #1097, .F. ) ;
#10174=ADVANCED_FACE ( 'NONE', ( #1957 ), #8126, .T. ) ;
#10179=ORIENTED_EDGE ( 'NONE', *, *, #7528, .F. ) ;
#10182=CARTESIAN_POINT ( 'NONE',  ( 203.2140370934807834, 48.77700970988914264, -0.9247215889056725757 ) ) ;
#10184=VERTEX_POINT ( 'NONE', #2280 ) ;
#10206=ORIENTED_EDGE ( 'NONE', *, *, #13336, .F. ) ;
#10215=CARTESIAN_POINT ( 'NONE',  ( 191.4227524587821279, 39.61567282607229856, -2.929995994935606252 ) ) ;
#10228=CARTESIAN_POINT ( 'NONE',  ( 188.3492591927541753, 42.47468418338397811, -7.638025320682917396 ) ) ;
#10274=CARTESIAN_POINT ( 'NONE',  ( 190.6753907620029054, 48.10438271498464502, -4.747728522856008659 ) ) ;
#10296=CARTESIAN_POINT ( 'NONE',  ( 162.8297652159045015, 17.20175482153034707, -6.370175303308202253 ) ) ;
#10305=CARTESIAN_POINT ( 'NONE',  ( 209.6520103264654438, 47.93571987055528183, -2.624305162434556582 ) ) ;
#10342=ORIENTED_EDGE ( 'NONE', *, *, #9312, .F. ) ;
#10352=AXIS2_PLACEMENT_3D ( 'NONE', #11333, #10078, #494 ) ;
#10354=CARTESIAN_POINT ( 'NONE',  ( 211.8867585259220050, 39.31811064754020890, -6.135149402309513000 ) ) ;
#10365=CARTESIAN_POINT ( 'NONE',  ( 194.7891036845171300, 47.85977741052224133, -6.433373108600371815 ) ) ;
#10381=CARTESIAN_POINT ( 'NONE',  ( 211.9051874564029561, 39.35763625820981559, -9.133132850359100274 ) ) ;
#10411=ADVANCED_FACE ( 'NONE', ( #4889 ), #3860, .T. ) ;
#10435=CARTESIAN_POINT ( 'NONE',  ( 204.0369835420791276, 51.66931235154874003, -2.492621690445610216 ) ) ;
#10459=CARTESIAN_POINT ( 'NONE',  ( 167.9295236634097819, 65.51901744756737855, -0.9107274384406879308 ) ) ;
#10462=CARTESIAN_POINT ( 'NONE',  ( 193.0268458394156710, 50.40397125358524733, -1.873914241081319210 ) ) ;
#10484=CARTESIAN_POINT ( 'NONE',  ( 154.0873337668446368, 6.722585725381706290, -7.588739505787663653 ) ) ;
#10487=ADVANCED_FACE ( 'NONE', ( #15418 ), #4490, .T. ) ;
#10530=CARTESIAN_POINT ( 'NONE',  ( 198.3593989614203963, 52.60648038231462920, -8.258707374242266752 ) ) ;
#10542=CARTESIAN_POINT ( 'NONE',  ( 194.8483215340629613, 47.90965193911861775, -4.864368187704507740 ) ) ;
#10588=CARTESIAN_POINT ( 'NONE',  ( 207.3822464892701305, 31.45897796630539744, -3.508361229271337312 ) ) ;
#10591=CIRCLE ( 'NONE', #13096, 1.500000000000000666 ) ;
#10617=CARTESIAN_POINT ( 'NONE',  ( 193.1446408943811548, 35.52021409135998198, -4.254410606405073736 ) ) ;
#10644=AXIS2_PLACEMENT_3D ( 'NONE', #8603, #123, #12289 ) ;
#10666=CARTESIAN_POINT ( 'NONE',  ( 209.5402858782260864, 48.07700032709870896, -2.761241636875660710 ) ) ;
#10688=VERTEX_POINT ( 'NONE', #12585 ) ;
#10694=CARTESIAN_POINT ( 'NONE',  ( 194.8602319459051557, 33.82038799488785230, -7.127215995405879134 ) ) ;
#10704=CARTESIAN_POINT ( 'NONE',  ( 198.9111841706756536, 32.15857605477618364, -5.308824953579920347 ) ) ;
#10722=DIRECTION ( 'NONE',  ( -1.000000000000000000, 0.000000000000000000, 0.000000000000000000 ) ) ;
#10743=ADVANCED_BREP_SHAPE_REPRESENTATION ( '', ( #642, #12337 ), #6298 ) ;
#10745=CARTESIAN_POINT ( 'NONE',  ( 191.4069380837317453, 39.61051162384328705, -7.503330758807070566 ) ) ;
#10746=SURFACE_STYLE_FILL_AREA ( #9333 ) ;
#10762=CARTESIAN_POINT ( 'NONE',  ( 170.9756796482968184, 59.36285257857151976, -0.9107274384406881529 ) ) ;
#10771=CARTESIAN_POINT ( 'NONE',  ( 201.9353358396146234, 32.56853033914327966, -9.715529407007519325 ) ) ;
#10782=CARTESIAN_POINT ( 'NONE',  ( 202.8187013049204950, 32.78779105710274422, -6.518094968334741779 ) ) ;
#10828=CARTESIAN_POINT ( 'NONE',  ( 198.9883150731717478, 32.15189384935130334, -6.877829860972676457 ) ) ;
#10830=FILL_AREA_STYLE_COLOUR ( '', #3569 ) ;
#10845=AXIS2_PLACEMENT_3D ( 'NONE', #8248, #5481, #4358 ) ;
#10856=CARTESIAN_POINT ( 'NONE',  ( 208.8253499713366352, 39.76173270276598970, -9.127040822819912691 ) ) ;
#10858=ORIENTED_EDGE ( 'NONE', *, *, #5334, .F. ) ;
#10861=CARTESIAN_POINT ( 'NONE',  ( 167.9295236634097819, 65.51901744756736434, -0.9107274384406985890 ) ) ;
#10867=CARTESIAN_POINT ( 'NONE',  ( 205.5168546899054434, 47.82311440310952833, -1.064259200291542529 ) ) ;
#10887=EDGE_CURVE ( 'NONE', #5154, #8651, #9573, .T. ) ;
#10905=MECHANICAL_DESIGN_GEOMETRIC_PRESENTATION_REPRESENTATION('',(#5592),#13920);
#10907=ORIENTED_EDGE ( 'NONE', *, *, #14756, .T. ) ;
#10908=CARTESIAN_POINT ( 'NONE',  ( 194.8335778941103626, 33.83376941343732369, -4.128887708184892702 ) ) ;
#10916=CARTESIAN_POINT ( 'NONE',  ( 202.6027916890166694, 29.64969172180087398, -8.171549047034778468 ) ) ;
#10933=CARTESIAN_POINT ( 'NONE',  ( 188.2949840871649485, 42.33905491644829766, -4.631930676406226688 ) ) ;
#10936=AXIS2_PLACEMENT_3D ( 'NONE', #6865, #4471, #9157 ) ;
#10943=CARTESIAN_POINT ( 'NONE',  ( 207.3546231538492179, 50.29643094772573164, -2.498001438440778710 ) ) ;
#10983=CARTESIAN_POINT ( 'NONE',  ( 201.3303440367248243, 32.15585396293944598, -6.755036635249508592 ) ) ;
#10985=VERTEX_POINT ( 'NONE', #10296 ) ;
#10989=CARTESIAN_POINT ( 'NONE',  ( 211.8984647248233273, 39.28052202550077965, -7.564127153369329726 ) ) ;
#10996=CARTESIAN_POINT ( 'NONE',  ( 163.3793289068652257, 15.80605437029538507, -6.370175303308196924 ) ) ;
#11007=CARTESIAN_POINT ( 'NONE',  ( 191.3918663844754349, 39.68659111044760124, -5.934329888686073140 ) ) ;
#11012=DIRECTION ( 'NONE',  ( -0.7900120431063429871, 0.6130913241491365850, 0.000000000000000000 ) ) ;
#11015=CARTESIAN_POINT ( 'NONE',  ( 192.8460887339186343, 31.43990810023382920, -3.998601258139535819 ) ) ;
#11022=ORIENTED_EDGE ( 'NONE', *, *, #14756, .F. ) ;
#11025=CARTESIAN_POINT ( 'NONE',  ( 208.8313558426846157, 41.97310978343666932, 0.1351797820921298021 ) ) ;
#11030=FACE_OUTER_BOUND ( 'NONE', #724, .T. ) ;
#11054=CARTESIAN_POINT ( 'NONE',  ( 201.2368453335255936, 49.57344380111126725, -8.378533376203868954 ) ) ;
#11059=VERTEX_POINT ( 'NONE', #10762 ) ;
#11062=CARTESIAN_POINT ( 'NONE',  ( 188.3116205180919565, 39.28179296801131670, -5.943714943518696003 ) ) ;
#11080=CYLINDRICAL_SURFACE ( 'NONE', #6040, 1.499999999999995115 ) ;
#11084=CARTESIAN_POINT ( 'NONE',  ( 208.8051451104704768, 39.65587490144260840, -4.559632177755815086 ) ) ;
#11094=CARTESIAN_POINT ( 'NONE',  ( 201.8058794277662571, 52.63602710067958412, -5.247041060177010330 ) ) ;
#11105=CARTESIAN_POINT ( 'NONE',  ( 191.4322133549729585, 42.19665789901188901, -4.493471110936619439 ) ) ;
#11119=DIRECTION ( 'NONE',  ( 0.9296197478520974444, 0.3660421972118351741, -0.04266420354037655377 ) ) ;
#11137=CARTESIAN_POINT ( 'NONE',  ( 208.8162124854775357, 42.04914431719598156, -1.433821094984975009 ) ) ;
#11143=CARTESIAN_POINT ( 'NONE',  ( 207.4378898283430885, 50.27467837972982068, -1.073754539701174959 ) ) ;
#11153=VERTEX_POINT ( 'NONE', #12169 ) ;
#11156=DIRECTION ( 'NONE',  ( -0.3663757939738424008, 0.9304669674900000187, 0.000000000000000000 ) ) ;
#11163=CARTESIAN_POINT ( 'NONE',  ( 207.0699012803337951, 46.20241706079673349, -2.754725152881798866 ) ) ;
#11174=CARTESIAN_POINT ( 'NONE',  ( 205.3747499027128924, 33.81850075496041796, -3.363818451488727934 ) ) ;
#11183=CARTESIAN_POINT ( 'NONE',  ( 198.8872864542346974, 32.16591232847088122, -2.310211674251309688 ) ) ;
#11212=CARTESIAN_POINT ( 'NONE',  ( 193.0950460371283839, 35.57958264137020876, -2.685405722344195389 ) ) ;
#11237=CARTESIAN_POINT ( 'NONE',  ( 191.4227524587821279, 39.61567282607229856, -2.929995994935606252 ) ) ;
#11239=CARTESIAN_POINT ( 'NONE',  ( 201.8629198063431716, 32.54887535240757757, -8.146526315903498627 ) ) ;
#11255=CARTESIAN_POINT ( 'NONE',  ( 205.5140042898306660, 47.80506208259531320, -5.491262609045910459 ) ) ;
#11282=CARTESIAN_POINT ( 'NONE',  ( 205.4319281802536068, 33.87189768065903905, -1.932853472788024440 ) ) ;
#11304=DIRECTION ( 'NONE',  ( 0.6130913241491353638, 0.7900120431063440973, -6.390853288715849130E-17 ) ) ;
#11308=CARTESIAN_POINT ( 'NONE',  ( 207.1164837741930569, 35.57719129110033407, -1.806778302941847159 ) ) ;
#11311=CARTESIAN_POINT ( 'NONE',  ( 198.8634854004546071, 49.55149448133588663, -6.680369717582868461 ) ) ;
#11328=CARTESIAN_POINT ( 'NONE',  ( 205.4727397017886119, 47.82775141623291404, -2.488642475836487566 ) ) ;
#11333=CARTESIAN_POINT ( 'NONE',  ( 170.6931741512129577, -3.595212766542494887, -13.46247879130521952 ) ) ;
#11367=CARTESIAN_POINT ( 'NONE',  ( 201.2658342953964166, 49.58143373454755931, -3.806719548689701416 ) ) ;
#11371=ORIENTED_EDGE ( 'NONE', *, *, #9692, .F. ) ;
#11394=CARTESIAN_POINT ( 'NONE',  ( 194.8381067511959372, 47.88228248201940573, -3.436395123936771601 ) ) ;
#11410=CARTESIAN_POINT ( 'NONE',  ( 190.5897039592268243, 47.97531786402677056, -7.885730391161881236 ) ) ;
#11434=CIRCLE ( 'NONE', #10936, 1.499999999999992228 ) ;
#11453=ORIENTED_EDGE ( 'NONE', *, *, #15575, .T. ) ;
#11463=CARTESIAN_POINT ( 'NONE',  ( 201.1780093772972009, 32.12620995903681376, -3.617034841014101776 ) ) ;
#11491=CARTESIAN_POINT ( 'NONE',  ( 190.6178699541428898, 33.66405957396897719, -4.118459193090428627 ) ) ;
#11535=CARTESIAN_POINT ( 'NONE',  ( 190.5897039592268243, 47.97531786402677056, -7.885730391161881236 ) ) ;
#11544=CARTESIAN_POINT ( 'NONE',  ( 207.1194509196011495, 46.14302886020001182, -1.185720282267065828 ) ) ;
#11563=CARTESIAN_POINT ( 'NONE',  ( 201.8058794277662571, 52.63602710067958412, -5.247041060177010330 ) ) ;
#11581=AXIS2_PLACEMENT_3D ( 'NONE', #10459, #15324, #4522 ) ;
#11609=ORIENTED_EDGE ( 'NONE', *, *, #7899, .T. ) ;
#11617=SHAPE_DEFINITION_REPRESENTATION ( #12541, #5419 ) ;
#11619=CARTESIAN_POINT ( 'NONE',  ( 188.3692075015854357, 39.10978640110493387, -4.508345083535985509 ) ) ;
#11624=CARTESIAN_POINT ( 'NONE',  ( 163.3793289068652257, 15.80605437029538507, -6.370175303308196924 ) ) ;
#11632=EDGE_LOOP ( 'NONE', ( #9188, #15172, #3690, #2301 ) ) ;
#11644=CYLINDRICAL_SURFACE ( 'NONE', #11581, 1.499999999999994227 ) ;
#11647=CARTESIAN_POINT ( 'NONE',  ( 204.3809113867051508, 51.54681031777401756, 0.6364305089822913652 ) ) ;
#11686=DIRECTION ( 'NONE',  ( 0.6130913241491352528, 0.7900120431063439863, -6.390853288715847897E-17 ) ) ;
#11724=CARTESIAN_POINT ( 'NONE',  ( 207.4341467637200651, 31.47497422714618764, -9.505705820141434614 ) ) ;
#11735=CARTESIAN_POINT ( 'NONE',  ( 194.8381067511959372, 47.88228248201940573, -3.436395123936771601 ) ) ;
#11772=CARTESIAN_POINT ( 'NONE',  ( 190.6749524420355328, 33.64372802412135144, -4.260924496400990691 ) ) ;
#11778=ORIENTED_EDGE ( 'NONE', *, *, #1290, .T. ) ;
#11797=CARTESIAN_POINT ( 'NONE',  ( 203.8319104552679448, 51.73948369304471839, -2.483607112462900446 ) ) ;
#11805=AXIS2_PLACEMENT_3D ( 'NONE', #11624, #6970, #4659 ) ;
#11810=CARTESIAN_POINT ( 'NONE',  ( 191.3767946852191528, 39.76267059705192253, -4.365329018565075714 ) ) ;
#11846=AXIS2_PLACEMENT_3D ( 'NONE', #8422, #3739, #9830 ) ;
#11852=CARTESIAN_POINT ( 'NONE',  ( 190.7182813446581235, 33.54593944905032998, -7.256469109801526152 ) ) ;
#11880=CARTESIAN_POINT ( 'NONE',  ( 207.3850704934720284, 31.45434786795649984, -6.508326106789642296 ) ) ;
#11888=CARTESIAN_POINT ( 'NONE',  ( 205.5140042898306660, 47.80506208259531320, -5.491262609045910459 ) ) ;
#11898=CARTESIAN_POINT ( 'NONE',  ( 205.4699394944333051, 33.88363592193200446, -7.930995773285529182 ) ) ;
#11917=DIRECTION ( 'NONE',  ( 0.6130913241491352528, 0.7900120431063439863, -6.390853288715847897E-17 ) ) ;
#11952=FACE_OUTER_BOUND ( 'NONE', #15145, .T. ) ;
#11956=CARTESIAN_POINT ( 'NONE',  ( 205.5291621427655002, 33.93354315402728361, -9.500001906449378808 ) ) ;
#11967=CARTESIAN_POINT ( 'NONE',  ( 203.2140370934807834, 48.77700970988914264, -0.9247215889056725757 ) ) ;
#11969=FACE_OUTER_BOUND ( 'NONE', #1102, .T. ) ;
#11975=CARTESIAN_POINT ( 'NONE',  ( 207.1325720688761294, 35.61275714886660637, -4.804596322733623914 ) ) ;
#12006=CARTESIAN_POINT ( 'NONE',  ( 201.3139613293953971, 49.56665511821758230, -6.809528532989353344 ) ) ;
#12007=( LENGTH_UNIT ( ) NAMED_UNIT ( * ) SI_UNIT ( .MILLI., .METRE. ) );
#12026=CARTESIAN_POINT ( 'NONE',  ( 209.6291075214908801, 33.76515323716659367, -3.385148507280513197 ) ) ;
#12035=CARTESIAN_POINT ( 'NONE',  ( 205.4339596421060889, 33.86846485884471747, -4.932823326473320336 ) ) ;
#12043=CARTESIAN_POINT ( 'NONE',  ( 194.7957337413261030, 33.86335648926068842, -5.558215102112974648 ) ) ;
#12046=ORIENTED_EDGE ( 'NONE', *, *, #7108, .F. ) ;
#12063=EDGE_CURVE ( 'NONE', #9626, #10985, #7964, .T. ) ;
#12076=CARTESIAN_POINT ( 'NONE',  ( 207.0793923465612352, 46.18607573428356972, -5.755770042397863051 ) ) ;
#12102=CARTESIAN_POINT ( 'NONE',  ( 208.8071490909987347, 39.71769555335276891, -3.129532392942456553 ) ) ;
#12112=CARTESIAN_POINT ( 'NONE',  ( 198.8340532681795594, 32.16525826020106393, -3.739820046187162905 ) ) ;
#12124=ORIENTED_EDGE ( 'NONE', *, *, #13336, .T. ) ;
#12133=DIRECTION ( 'NONE',  ( -1.000000000000000000, 0.000000000000000000, 0.000000000000000000 ) ) ;
#12161=CARTESIAN_POINT ( 'NONE',  ( 207.3258607540788319, 31.40438376407220389, -4.939321231805051227 ) ) ;
#12169=CARTESIAN_POINT ( 'NONE',  ( 151.6469155423420716, 8.238904255104483099, -6.725526318947268045 ) ) ;
#12186=CARTESIAN_POINT ( 'NONE',  ( 188.3378656401271201, 39.26133998289535043, -1.370343197488200548 ) ) ;
#12194=CARTESIAN_POINT ( 'NONE',  ( 193.1249951165660548, 46.22013307728793308, -3.310989833511668756 ) ) ;
#12196=ORIENTED_EDGE ( 'NONE', *, *, #3880, .T. ) ;
#12234=CARTESIAN_POINT ( 'NONE',  ( 188.3564733894159815, 42.55163899863504184, -6.069020498571065403 ) ) ;
#12253=CARTESIAN_POINT ( 'NONE',  ( 201.2541767070109984, 32.14103196098812987, -5.186035738131804962 ) ) ;
#12261=CARTESIAN_POINT ( 'NONE',  ( 205.4727397017886119, 47.82775141623291404, -2.488642475836487566 ) ) ;
#12270=CARTESIAN_POINT ( 'NONE',  ( 207.1663125311009992, 46.09156421935289671, -5.616260741029326375 ) ) ;
#12272=EDGE_LOOP ( 'NONE', ( #10161, #9047, #9044, #3964, #277 ) ) ;
#12274=CARTESIAN_POINT ( 'NONE',  ( 170.6931741512129577, -3.595212766542494887, -13.46247879130521952 ) ) ;
#12283=DIRECTION ( 'NONE',  ( -0.000000000000000000, -1.000000000000000000, -0.000000000000000000 ) ) ;
#12289=DIRECTION ( 'NONE',  ( -0.2258817899775119320, -0.9741547192086866813, 0.000000000000000000 ) ) ;
#12310=CARTESIAN_POINT ( 'NONE',  ( 203.1913894652216186, 29.76335179383669782, -8.124653964949581919 ) ) ;
#12323=CARTESIAN_POINT ( 'NONE',  ( 163.3793289068652541, 15.80605437029534954, -6.370175303308202253 ) ) ;
#12331=CARTESIAN_POINT ( 'NONE',  ( 205.4496313998743915, 47.84832575209421890, -7.060263518810960370 ) ) ;
#12337=AXIS2_PLACEMENT_3D ( 'NONE', #4568, #8147, #5681 ) ;
#12341=CARTESIAN_POINT ( 'NONE',  ( 202.9867918041427686, 48.86553571320913392, 0.6621522355815065985 ) ) ;
#12352=CARTESIAN_POINT ( 'NONE',  ( 205.3747499027128924, 33.81850075496041796, -3.363818451488727934 ) ) ;
#12390=CARTESIAN_POINT ( 'NONE',  ( 192.9674079352396348, 50.35451258660443585, -3.442919105360563226 ) ) ;
#12410=DIRECTION ( 'NONE',  ( 0.6130913241491352528, 0.7900120431063439863, -6.390853288732736916E-17 ) ) ;
#12411=CARTESIAN_POINT ( 'NONE',  ( 207.1131222881253393, 35.56952893079440514, -7.807171136772324438 ) ) ;
#12417=CARTESIAN_POINT ( 'NONE',  ( 165.4217645774054120, 62.57671370024034729, -0.9107274384406883749 ) ) ;
#12418=ADVANCED_FACE ( 'NONE', ( #152 ), #6261, .T. ) ;
#12426=CARTESIAN_POINT ( 'NONE',  ( 193.1436046380909772, 46.22450523326372007, -4.738359826975481859 ) ) ;
#12459=CARTESIAN_POINT ( 'NONE',  ( 205.5168546899054434, 47.82311440310952833, -1.064259200291542529 ) ) ;
#12483=CARTESIAN_POINT ( 'NONE',  ( 202.3883256910358739, 32.65987148549056229, -8.116337980372584582 ) ) ;
#12499=ORIENTED_EDGE ( 'NONE', *, *, #9312, .T. ) ;
#12501=CARTESIAN_POINT ( 'NONE',  ( 207.1194509196011495, 46.14302886020001182, -1.185720282267065828 ) ) ;
#12518=DIRECTION ( 'NONE',  ( 0.000000000000000000, 0.000000000000000000, -1.000000000000000000 ) ) ;
#12541=PRODUCT_DEFINITION_SHAPE ( 'NONE', 'NONE',  #6143 ) ;
#12574=CARTESIAN_POINT ( 'NONE',  ( 188.3636875860777593, 42.62859381388609137, -4.500015676459212521 ) ) ;
#12585=CARTESIAN_POINT ( 'NONE',  ( 170.9049199631132581, 71.79964605558720336, -0.9107274384406883749 ) ) ;
#12605=AXIS2_PLACEMENT_3D ( 'NONE', #10157, #3984, #1851 ) ;
#12616=CARTESIAN_POINT ( 'NONE',  ( 194.8381067511959372, 47.88228248201940573, -3.436395123936771601 ) ) ;
#12633=CARTESIAN_POINT ( 'NONE',  ( 208.8313558426846157, 41.97310978343666932, 0.1351797820921298021 ) ) ;
#12640=ORIENTED_EDGE ( 'NONE', *, *, #3183, .F. ) ;
#12644=CARTESIAN_POINT ( 'NONE',  ( 193.0950460371283839, 35.57958264137020876, -2.685405722344195389 ) ) ;
#12657=CARTESIAN_POINT ( 'NONE',  ( 190.7182813446581235, 33.54593944905032998, -7.256469109801526152 ) ) ;
#12706=CARTESIAN_POINT ( 'NONE',  ( 209.6240687314160880, 33.75364762868482416, -9.385773361654676350 ) ) ;
#12717=CARTESIAN_POINT ( 'NONE',  ( 201.3139613293953971, 49.56665511821758230, -6.809528532989353344 ) ) ;
#12723=DIRECTION ( 'NONE',  ( 0.9296197478520975555, 0.3660421972118350631, -0.04266420354037653295 ) ) ;
#12733=CARTESIAN_POINT ( 'NONE',  ( 209.5435894037482285, 33.63601521402413397, -0.2471466635189603911 ) ) ;
#12749=DIRECTION ( 'NONE',  ( 0.6130913241491352528, 0.7900120431063439863, -6.390853288715847897E-17 ) ) ;
#12781=CARTESIAN_POINT ( 'NONE',  ( 203.9349922441545857, 30.00251698353133989, -9.664403529890410738 ) ) ;
#12810=CARTESIAN_POINT ( 'NONE',  ( 202.4110361843541455, 29.59410989755560806, -6.585651355106874050 ) ) ;
#12828=DIRECTION ( 'NONE',  ( -0.8204839007831782327, 0.5707893219124419160, -0.03171306586179808984 ) ) ;
#12865=CARTESIAN_POINT ( 'NONE',  ( 209.6393851568315938, 47.95822392590527983, 0.3767681043515945238 ) ) ;
#12894=CARTESIAN_POINT ( 'NONE',  ( 188.3076603040395582, 42.49356297222218615, -1.493920802967548367 ) ) ;
#12899=CARTESIAN_POINT ( 'NONE',  ( 162.8297652159045015, 17.20175482153035063, -6.370175303308202253 ) ) ;
#12942=CARTESIAN_POINT ( 'NONE',  ( 209.5531742284681798, 48.05466962632709027, -5.762314779011898480 ) ) ;
#12956=EDGE_CURVE ( 'NONE', #5373, #10184, #11434, .T. ) ;
#12970=CARTESIAN_POINT ( 'NONE',  ( 201.2368453335255936, 49.57344380111126725, -8.378533376203868954 ) ) ;
#12979=CARTESIAN_POINT ( 'NONE',  ( 201.3139613293953971, 49.56665511821758230, -6.809528532989353344 ) ) ;
#13014=CARTESIAN_POINT ( 'NONE',  ( 202.5558682508970492, 29.63341987102701580, -9.723657537314917221 ) ) ;
#13035=CARTESIAN_POINT ( 'NONE',  ( 194.7786688470199010, 47.83282381504752578, -5.005399988216014506 ) ) ;
#13046=CARTESIAN_POINT ( 'NONE',  ( 191.3844089520862894, 42.02011290432638901, -3.056456915890917170 ) ) ;
#13053=CARTESIAN_POINT ( 'NONE',  ( 193.1265229109121435, 35.50728864820005981, -5.680987958736793075 ) ) ;
#13092=CARTESIAN_POINT ( 'NONE',  ( 202.8882743124338504, 32.81631024066724933, -8.087096619718394663 ) ) ;
#13096=AXIS2_PLACEMENT_3D ( 'NONE', #10061, #5401, #13675 ) ;
#13115=AXIS2_PLACEMENT_3D ( 'NONE', #7490, #12283, #12518 ) ;
#13121=CARTESIAN_POINT ( 'NONE',  ( 207.3822464892701305, 31.45897796630539744, -3.508361229271337312 ) ) ;
#13130=CARTESIAN_POINT ( 'NONE',  ( 207.1164837741930569, 35.57719129110033407, -1.806778302941847159 ) ) ;
#13165=AXIS2_PLACEMENT_3D ( 'NONE', #9630, #7350, #3623 ) ;
#13170=CARTESIAN_POINT ( 'NONE',  ( 207.1750190499664370, 35.67744599754978907, -6.373597270514506974 ) ) ;
#13186=AXIS2_PLACEMENT_3D ( 'NONE', #5494, #9207, #15252 ) ;
#13190=DIRECTION ( 'NONE',  ( -0.9741547192086867923, 0.2258817899775114602, 0.000000000000000000 ) ) ;
#13194=CARTESIAN_POINT ( 'NONE',  ( 208.7972876766878016, 42.12791357830437988, -6.002605234521809052 ) ) ;
#13195=AXIS2_PLACEMENT_3D ( 'NONE', #8517, #9620, #1231 ) ;
#13208=CARTESIAN_POINT ( 'NONE',  ( 201.2658342953964166, 49.58143373454755931, -3.806719548689701416 ) ) ;
#13216=CARTESIAN_POINT ( 'NONE',  ( 191.3918663844754349, 39.68659111044760124, -5.934329888686073140 ) ) ;
#13232=CARTESIAN_POINT ( 'NONE',  ( 163.9288925978260352, 14.41035391906035201, -6.370175303308202253 ) ) ;
#13235=( LENGTH_UNIT ( ) NAMED_UNIT ( * ) SI_UNIT ( .MILLI., .METRE. ) );
#13274=CARTESIAN_POINT ( 'NONE',  ( 190.6221111713484788, 48.05726534264031358, -4.889407597981446862 ) ) ;
#13282=CARTESIAN_POINT ( 'NONE',  ( 207.1690005588685040, 46.08364065960329725, 0.3832845883476674320 ) ) ;
#13291=B_SPLINE_CURVE_WITH_KNOTS ( 'NONE', 3,
 ( #11239, #3450, #8281, #11898, #8878, #8958, #4121, #5477, #3027, #12717, #11311, #10365, #6672, #4354, #13989, #4270, #9189, #5395, #9031, #1906, #7933, #13829, #15082, #6818, #7771, #5552, #471, #11394, #1752, #7858, #10215, #12644, #6744, #4044, #4192, #557, #5313, #13670, #3176, #11544, #709, #10056, #9113, #15159 ),
 .UNSPECIFIED., .F., .F.,
 ( 4, 2, 2, 2, 2, 2, 2, 2, 2, 2, 2, 2, 2, 2, 2, 2, 2, 2, 2, 2, 2, 4 ),
 ( 0.000000000000000000, 0.01154246058414762008, 0.06319472280952896648, 0.1156547325041140800, 0.1678637871092111822, 0.2189476930995808979, 0.2714221776790743945, 0.3227197530690046334, 0.3747274728241424824, 0.4267432521036158555, 0.4780248536244998681, 0.5305055628088307662, 0.5815973485975094448, 0.6337991395759137170, 0.6855599279679012170, 0.7371634071600560167, 0.7894711232639126663, 0.8405207634104210346, 0.8929453349049019106, 0.9452650328228678900, 0.9965476795071586125, 1.000000000000000000 ),
 .UNSPECIFIED. ) ;
#13327=CARTESIAN_POINT ( 'NONE',  ( 208.8071490909987347, 39.71769555335276891, -3.129532392942456553 ) ) ;
#13333=CARTESIAN_POINT ( 'NONE',  ( 207.3463650020273974, 50.30900816961851518, -7.069655767765518739 ) ) ;
#13336=EDGE_CURVE ( 'NONE', #9376, #11059, #13955, .T. ) ;
#13368=CARTESIAN_POINT ( 'NONE',  ( 194.8975446553719451, 47.93174114899129989, -1.867390259657528251 ) ) ;
#13376=CARTESIAN_POINT ( 'NONE',  ( 193.1007612367029367, 46.15997280778478995, -6.307360761128419036 ) ) ;
#13380=ADVANCED_FACE ( 'NONE', ( #1081 ), #329, .T. ) ;
#13383=DIRECTION ( 'NONE',  ( -0.9741547192086867923, 0.2258817899775115157, 1.688901894271609290E-28 ) ) ;
#13410=CARTESIAN_POINT ( 'NONE',  ( 201.8629198063431716, 32.54887535240757757, -8.146526315903498627 ) ) ;
#13445=CARTESIAN_POINT ( 'NONE',  ( 205.5810540386909508, 47.77928077683765906, 0.5047415929677595559 ) ) ;
#13454=CARTESIAN_POINT ( 'NONE',  ( 203.2853005557455788, 48.75346994511389198, 0.6442813861133344089 ) ) ;
#13489=CARTESIAN_POINT ( 'NONE',  ( 201.6633919852714030, 52.66288709485617403, -3.813211015790380909 ) ) ;
#13509=CARTESIAN_POINT ( 'NONE',  ( 207.1325720688761294, 35.61275714886660637, -4.804596322733623914 ) ) ;
#13519=CARTESIAN_POINT ( 'NONE',  ( 198.9622538275367845, 49.57425033952682014, -2.112703922695001513 ) ) ;
#13527=CARTESIAN_POINT ( 'NONE',  ( 207.0703735592109069, 35.50494473061488065, -6.238171316985951620 ) ) ;
#13564=CARTESIAN_POINT ( 'NONE',  ( 198.4664250651615021, 52.63210452169714415, -3.691074174585086798 ) ) ;
#13572=( NAMED_UNIT ( * ) PLANE_ANGLE_UNIT ( ) SI_UNIT ( $, .RADIAN. ) );
#13588=CARTESIAN_POINT ( 'NONE',  ( 208.8002188652075972, 39.64064887424692785, -1.560527519332197022 ) ) ;
#13598=ORIENTED_EDGE ( 'NONE', *, *, #229, .T. ) ;
#13608=CARTESIAN_POINT ( 'NONE',  ( 208.8162124854775357, 42.04914431719598156, -1.433821094984975009 ) ) ;
#13662=CLOSED_SHELL ( 'NONE', ( #7038, #13380, #13757, #12418, #10487, #15146, #8191, #15318, #13936, #3054, #9618, #5162, #10174, #10411, #491, #15453 ) ) ;
#13668=CARTESIAN_POINT ( 'NONE',  ( 202.8426534586648700, 48.90729187601812811, -2.475854291071949209 ) ) ;
#13670=CARTESIAN_POINT ( 'NONE',  ( 208.8002188652075972, 39.64064887424692785, -1.560527519332197022 ) ) ;
#13675=DIRECTION ( 'NONE',  ( -0.3662838836490099337, 0.9305003370641709015, 0.002288952263120960697 ) ) ;
#13686=CARTESIAN_POINT ( 'NONE',  ( 208.7983505906672121, 39.57879239708907448, -2.990627279509298742 ) ) ;
#13757=ADVANCED_FACE ( 'NONE', ( #14104 ), #9286, .T. ) ;
#13767=CARTESIAN_POINT ( 'NONE',  ( 205.3727474927790411, 33.82195144205066839, -0.3638485434072702973 ) ) ;
#13795=CARTESIAN_POINT ( 'NONE',  ( 198.8863654052626657, 49.55881746625484396, -3.681704842056328086 ) ) ;
#13814=CARTESIAN_POINT ( 'NONE',  ( 207.4107378919655673, 50.26574450011962369, -5.500654858001599479 ) ) ;
#13815=DIRECTION ( 'NONE',  ( 0.9296197478520974444, 0.3660421972118351741, -0.04266420354037655377 ) ) ;
#13829=CARTESIAN_POINT ( 'NONE',  ( 208.8051451104704768, 39.65587490144260840, -4.559632177755815086 ) ) ;
#13846=CARTESIAN_POINT ( 'NONE',  ( 204.1803465669382547, 51.62486026858844212, 0.6453845751958426913 ) ) ;
#13860=CIRCLE ( 'NONE', #10845, 6.299128011492294732 ) ;
#13901=CARTESIAN_POINT ( 'NONE',  ( 203.9760488007458719, 51.69772753023573131, 0.6543994141905550288 ) ) ;
#13920=( GEOMETRIC_REPRESENTATION_CONTEXT ( 3 ) GLOBAL_UNCERTAINTY_ASSIGNED_CONTEXT ( ( #8022 ) ) GLOBAL_UNIT_ASSIGNED_CONTEXT ( ( #12007, #13572, #9483 ) ) REPRESENTATION_CONTEXT ( 'NONE', 'WORKASPACE' ) );
#13922=EDGE_LOOP ( 'NONE', ( #1320, #1421, #10206, #2780 ) ) ;
#13929=CARTESIAN_POINT ( 'NONE',  ( 190.7088546992480076, 48.18597428004899541, -1.751405883087224113 ) ) ;
#13936=ADVANCED_FACE ( 'NONE', ( #4182 ), #2785, .T. ) ;
#13955=CIRCLE ( 'NONE', #13195, 1.499999999999995115 ) ;
#13979=CARTESIAN_POINT ( 'NONE',  ( 190.6221111713484788, 48.05726534264031358, -4.889407597981446862 ) ) ;
#13989=CARTESIAN_POINT ( 'NONE',  ( 191.3918663844754349, 39.68659111044760124, -5.934329888686073140 ) ) ;
#13998=CARTESIAN_POINT ( 'NONE',  ( 203.4093511297053851, 50.30250970312692971, -0.9107274384406970347 ) ) ;
#14002=CARTESIAN_POINT ( 'NONE',  ( 192.9750851430037528, 31.35397111148814631, -7.136603044727629630 ) ) ;
#14047=CARTESIAN_POINT ( 'NONE',  ( 201.5861714792528119, 52.66925088518574682, -5.382215963875594866 ) ) ;
#14076=CARTESIAN_POINT ( 'NONE',  ( 202.9867918041427686, 48.86553571320913392, 0.6621522355815065985 ) ) ;
#14104=FACE_OUTER_BOUND ( 'NONE', #9185, .T. ) ;
#14155=CARTESIAN_POINT ( 'NONE',  ( 203.9349922441545857, 30.00251698353133989, -9.664403529890410738 ) ) ;
#14163=CARTESIAN_POINT ( 'NONE',  ( 207.1194509196011495, 46.14302886020001182, -1.185720282267065828 ) ) ;
#14169=CARTESIAN_POINT ( 'NONE',  ( 152.8671246545933400, 7.480744990243093362, -7.157132912367466737 ) ) ;
#14183=CIRCLE ( 'NONE', #3634, 1.499999999999994227 ) ;
#14187=VERTEX_POINT ( 'NONE', #4801 ) ;
#14195=CARTESIAN_POINT ( 'NONE',  ( 167.9295236634097819, 65.51901744756736434, -0.9107274384406985890 ) ) ;
#14202=CARTESIAN_POINT ( 'NONE',  ( 211.8802283582561472, 39.29745248741442509, -3.136047433260559902 ) ) ;
#14229=CARTESIAN_POINT ( 'NONE',  ( 201.5861714792528119, 52.66925088518574682, -5.382215963875594866 ) ) ;
#14241=CARTESIAN_POINT ( 'NONE',  ( 194.7891036845171300, 47.85977741052224133, -6.433373108600371815 ) ) ;
#14247=CARTESIAN_POINT ( 'NONE',  ( 205.4699394944333051, 33.88363592193200446, -7.930995773285529182 ) ) ;
#14252=VERTEX_POINT ( 'NONE', #1386 ) ;
#14270=DIRECTION ( 'NONE',  ( -1.000000000000000000, 0.000000000000000000, 0.000000000000000000 ) ) ;
#14277=CARTESIAN_POINT ( 'NONE',  ( 191.4384233894935505, 39.53989603517709384, -4.498996937958945175 ) ) ;
#14301=CARTESIAN_POINT ( 'NONE',  ( 191.4384233894935505, 39.53989603517709384, -4.498996937958945175 ) ) ;
#14310=CIRCLE ( 'NONE', #11805, 1.500000000000000666 ) ;
#14314=CARTESIAN_POINT ( 'NONE',  ( 202.3171501287270644, 32.63561614260228794, -6.547335233887139339 ) ) ;
#14326=CARTESIAN_POINT ( 'NONE',  ( 207.0699012803337951, 46.20241706079673349, -2.754725152881798866 ) ) ;
#14358=CARTESIAN_POINT ( 'NONE',  ( 207.1167095084715868, 46.15093117762712893, -7.185265714380067337 ) ) ;
#14385=CARTESIAN_POINT ( 'NONE',  ( 204.2383844621755884, 51.59388984732451888, -2.501575441055724713 ) ) ;
#14395=CARTESIAN_POINT ( 'NONE',  ( 207.1288103955774318, 46.12660085639766550, -4.186765234109192768 ) ) ;
#14419=ORIENTED_EDGE ( 'NONE', *, *, #7899, .F. ) ;
#14420=( NAMED_UNIT ( * ) SI_UNIT ( $, .STERADIAN. ) SOLID_ANGLE_UNIT ( ) );
#14436=CARTESIAN_POINT ( 'NONE',  ( 205.4911088677281725, 33.92184391926740972, -3.501858402168778639 ) ) ;
#14462=CARTESIAN_POINT ( 'NONE',  ( 202.9578473199472057, 32.84482942423175444, -9.656098271102047548 ) ) ;
#14471=CARTESIAN_POINT ( 'NONE',  ( 201.7905037730716913, 32.52922036567187547, -6.577523224799477930 ) ) ;
#14512=CARTESIAN_POINT ( 'NONE',  ( 205.4526553411199359, 47.86694802938139759, -2.633259993550844502 ) ) ;
#14520=CARTESIAN_POINT ( 'NONE',  ( 211.8897246948783106, 42.46053108337658699, -4.442978748809460754 ) ) ;
#14537=CARTESIAN_POINT ( 'NONE',  ( 198.9111841706756536, 32.15857605477618364, -5.308824953579920347 ) ) ;
#14544=CARTESIAN_POINT ( 'NONE',  ( 201.5722569949026877, 29.04292258031605556, -3.626438834624695406 ) ) ;
#14589=CARTESIAN_POINT ( 'NONE',  ( 191.3780708436489704, 41.94285887643944477, -4.625461852610818880 ) ) ;
#14597=CARTESIAN_POINT ( 'NONE',  ( 190.6325473606148648, 48.03985028950570779, -6.316729457008944948 ) ) ;
#14619=CARTESIAN_POINT ( 'NONE',  ( 203.0658429208174880, 48.83360436048501896, -0.9158339742359169477 ) ) ;
#14633=CARTESIAN_POINT ( 'NONE',  ( 198.8102040144913758, 32.17279782253822162, -0.7412068558913099681 ) ) ;
#14641=CARTESIAN_POINT ( 'NONE',  ( 208.8119045081773777, 39.60750423734790360, -5.989029428842635561 ) ) ;
#14669=CARTESIAN_POINT ( 'NONE',  ( 194.7691866843436799, 33.87697957786221536, -2.559886773443665220 ) ) ;
#14677=CARTESIAN_POINT ( 'NONE',  ( 203.8654192366412587, 29.97399779996683833, -8.095401878506494953 ) ) ;
#14683=ORIENTED_EDGE ( 'NONE', *, *, #15575, .F. ) ;
#14689=DIRECTION ( 'NONE',  ( -0.3663757939738424008, 0.9304669674900000187, 0.000000000000000000 ) ) ;
#14695=CARTESIAN_POINT ( 'NONE',  ( 198.8634854004546071, 49.55149448133588663, -6.680369717582868461 ) ) ;
#14703=CARTESIAN_POINT ( 'NONE',  ( 188.3636875860777593, 42.62859381388609137, -4.500015676459212521 ) ) ;
#14704=ORIENTED_EDGE ( 'NONE', *, *, #2388, .T. ) ;
#14714=CARTESIAN_POINT ( 'NONE',  ( 198.8863654052626657, 49.55881746625484396, -3.681704842056328086 ) ) ;
#14744=CARTESIAN_POINT ( 'NONE',  ( 198.8872864542346974, 32.16591232847088122, -2.310211674251309688 ) ) ;
#14756=EDGE_CURVE ( 'NONE', #5773, #9626, #15586, .T. ) ;
#14771=CARTESIAN_POINT ( 'NONE',  ( 194.8381067511959372, 47.88228248201940573, -3.436395123936771601 ) ) ;
#14785=CARTESIAN_POINT ( 'NONE',  ( 205.4319281802536068, 33.87189768065903905, -1.932853472788024440 ) ) ;
#14846=CARTESIAN_POINT ( 'NONE',  ( 193.1249951165660548, 46.22013307728793308, -3.310989833511668756 ) ) ;
#14865=CARTESIAN_POINT ( 'NONE',  ( 193.0454511798755846, 35.63895119138042133, -1.116400838283317043 ) ) ;
#14899=CARTESIAN_POINT ( 'NONE',  ( 202.9147226314038051, 48.88641379461363101, -0.9068510277452211943 ) ) ;
#14923=DIRECTION ( 'NONE',  ( -0.7900120431063439863, 0.6130913241491352528, 0.000000000000000000 ) ) ;
#14934=B_SPLINE_SURFACE_WITH_KNOTS ( 'NONE', 3, 3, ( 
 ( #4624, #103, #6058, #14247, #2341, #8278, #983, #5892, #3446, #4944, #30, #8584, #13376, #8437, #13216, #13053, #12043, #2256, #1216, #15502, #11975, #1145, #5972, #4135, #1449, #8661, #14714, #5175, #12194, #9923, #2730, #6372, #8733, #11183, #10002, #14785, #7474, #5328, #13608, #12501, #10072, #8897, #5022, #258 ),
 ( #5099, #10153, #2813, #3910, #13527, #14641, #2892, #12270, #11255, #7553, #334, #6286, #12426, #11105, #1618, #3978, #8810, #6528, #7635, #12352, #6449, #13686, #2965, #7715, #11328, #1374, #1535, #410, #14945, #5247, #8974, #14865, #1692, #4061, #489, #13767, #6212, #3839, #11025, #174, #9849, #13454, #2653, #14076 ),
 ( #12810, #4526, #5491, #3270, #9046, #9129, #15097, #5570, #7949, #11563, #4446, #5643, #887, #12574, #809, #11491, #4289, #1844, #8111, #1771, #15327, #6914, #4369, #10305, #575, #5412, #1999, #10462, #13929, #12894, #6757, #4209, #3118, #7791, #6837, #2080, #12733, #651, #6688, #1921, #15250, #11647, #13846, #9279 ),
 ( #3045, #7874, #14155, #11724, #5719, #10381, #15174, #9356, #6606, #727, #10530, #9205, #11410, #10228, #15022, #12657, #14002, #3192, #8023, #11880, #6114, #7232, #1128, #15485, #4928, #14229, #2397, #4849, #13274, #10933, #4762, #9585, #5950, #3350, #3501, #13121, #12026, #1195, #4680, #3583, #7070, #14385, #9745, #11797 ),
 ( #10771, #6034, #14462, #11956, #1052, #10856, #3427, #8336, #8187, #12970, #88, #2157, #7150, #4607, #9430, #2321, #10694, #5876, #6992, #11, #8260, #8418, #13194, #9508, #3656, #1282, #965, #13035, #2236, #5793, #14301, #10617, #15557, #9667, #8492, #2470, #7304, #12102, #15407, #11163, #8876, #2873, #8791, #13668 ),
 ( #7694, #12483, #8717, #6354, #12411, #9985, #8561, #317, #12331, #6195, #14695, #8639, #6509, #3819, #11007, #1433, #7534, #14537, #12253, #5080, #13509, #11084, #2712, #1517, #5157, #9825, #1675, #14771, #14846, #1595, #11237, #7386, #2635, #393, #3963, #7457, #11308, #13588, #6269, #237, #1356, #5231, #14619, #2793 ) ),
 .UNSPECIFIED., .T., .F., .F.,
 ( 4, 2, 4 ),
 ( 4, 2, 2, 2, 2, 2, 2, 2, 2, 2, 2, 2, 2, 2, 2, 2, 2, 2, 2, 2, 2, 4 ),
 ( 0.000000000000000000, 0.5000000000000000000, 1.000000000000000000 ),
 ( 0.000000000000000000, 0.01154246058414762008, 0.06319472280952896648, 0.1156547325041140800, 0.1678637871092111822, 0.2189476930995808979, 0.2714221776790743945, 0.3227197530690046334, 0.3747274728241424824, 0.4267432521036158555, 0.4780248536244998681, 0.5305055628088307662, 0.5815973485975094448, 0.6337991395759137170, 0.6855599279679012170, 0.7371634071600560167, 0.7894711232639126663, 0.8405207634104210346, 0.8929453349049019106, 0.9452650328228678900, 0.9965476795071586125, 1.000000000000000000 ),
 .UNSPECIFIED. ) ;
#14945=CARTESIAN_POINT ( 'NONE',  ( 193.1683668805158334, 46.28448754599228465, -1.741988976065122152 ) ) ;
#14992=CARTESIAN_POINT ( 'NONE',  ( 209.5385712735872517, 33.62447922832576097, -6.247773722084159154 ) ) ;
#15022=CARTESIAN_POINT ( 'NONE',  ( 188.3266922173125124, 39.20571348140700252, -7.512715813640810758 ) ) ;
#15067=PRODUCT_CONTEXT ( 'NONE', #3521, 'mechanical' ) ;
#15069=CARTESIAN_POINT ( 'NONE',  ( 190.6178699541428898, 33.66405957396897719, -4.118459193090428627 ) ) ;
#15071=ORIENTED_EDGE ( 'NONE', *, *, #12063, .F. ) ;
#15082=CARTESIAN_POINT ( 'NONE',  ( 208.8124460758720033, 42.05191026284237665, -4.433604294307299298 ) ) ;
#15087=AXIS2_PLACEMENT_3D ( 'NONE', #3227, #11686, #5607 ) ;
#15097=CARTESIAN_POINT ( 'NONE',  ( 211.8964099132376191, 42.41229301046570299, -5.872780407435223893 ) ) ;
#15145=EDGE_LOOP ( 'NONE', ( #4905, #12196, #2146, #5851 ) ) ;
#15146=ADVANCED_FACE ( 'NONE', ( #11952 ), #11644, .T. ) ;
#15149=CARTESIAN_POINT ( 'NONE',  ( 207.2255354594468884, 50.38222520613008015, -5.636003230111601425 ) ) ;
#15159=CARTESIAN_POINT ( 'NONE',  ( 202.9928097691983169, 48.86380790798758511, -0.9029304599467440351 ) ) ;
#15172=ORIENTED_EDGE ( 'NONE', *, *, #6163, .T. ) ;
#15174=CARTESIAN_POINT ( 'NONE',  ( 211.8657363685815653, 42.56416725473636831, -9.010781945348840694 ) ) ;
#15180=EDGE_CURVE ( 'NONE', #10184, #5373, #4769, .T. ) ;
#15226=CARTESIAN_POINT ( 'NONE',  ( 201.8412736707888087, 29.11599755995149152, -3.759251452247287517 ) ) ;
#15250=CARTESIAN_POINT ( 'NONE',  ( 207.5020891771285960, 50.23084475345794431, 0.4952462535581279024 ) ) ;
#15252=DIRECTION ( 'NONE',  ( -0.3662838836490107108, 0.9305003370641705684, 0.002288952263120965468 ) ) ;
#15294=DIRECTION ( 'NONE',  ( -1.000000000000000000, 0.000000000000000000, 0.000000000000000000 ) ) ;
#15298=CARTESIAN_POINT ( 'NONE',  ( 201.7245916543302826, 29.07256658421868423, -6.764440628860102223 ) ) ;
#15318=ADVANCED_FACE ( 'NONE', ( #8635 ), #11080, .T. ) ;
#15324=DIRECTION ( 'NONE',  ( 0.6130913241491352528, 0.7900120431063440973, -6.390853288732736916E-17 ) ) ;
#15327=CARTESIAN_POINT ( 'NONE',  ( 209.5657782771801578, 33.68426770849990959, -3.244931658323684687 ) ) ;
#15337=CARTESIAN_POINT ( 'NONE',  ( 193.1436046380909772, 46.22450523326372007, -4.738359826975481859 ) ) ;
#15363=AXIS2_PLACEMENT_3D ( 'NONE', #9032, #13383, #1754 ) ;
#15373=DIRECTION ( 'NONE',  ( 0.6130913241491352528, 0.7900120431063439863, -6.390853288732736916E-17 ) ) ;
#15387=ORIENTED_EDGE ( 'NONE', *, *, #4376, .T. ) ;
#15407=CARTESIAN_POINT ( 'NONE',  ( 208.8010691282704840, 42.12517885095529380, -3.002821972062079681 ) ) ;
#15416=EDGE_LOOP ( 'NONE', ( #5567, #12124, #13598, #3112 ) ) ;
#15418=FACE_OUTER_BOUND ( 'NONE', #1901, .T. ) ;
#15443=ORIENTED_EDGE ( 'NONE', *, *, #1290, .F. ) ;
#15453=ADVANCED_FACE ( 'NONE', ( #2869 ), #8872, .T. ) ;
#15458=CARTESIAN_POINT ( 'NONE',  ( 204.2383844621755884, 51.59388984732451888, -2.501575441055724713 ) ) ;
#15485=CARTESIAN_POINT ( 'NONE',  ( 209.5531742284681798, 48.05466962632709027, -5.762314779011898480 ) ) ;
#15496=CARTESIAN_POINT ( 'NONE',  ( 202.9147226314038051, 48.88641379461363101, -0.9068510277452211943 ) ) ;
#15502=CARTESIAN_POINT ( 'NONE',  ( 205.4339596421060889, 33.86846485884471747, -4.932823326473320336 ) ) ;
#15530=CARTESIAN_POINT ( 'NONE',  ( 194.8602319459051557, 33.82038799488785230, -7.127215995405879134 ) ) ;
#15542=B_SPLINE_CURVE_WITH_KNOTS ( 'NONE', 3,
 ( #10916, #12310, #14677, #8542, #1413, #10989, #8855, #6177, #13333, #3797, #9885, #1261, #14597, #12234, #11062, #6249, #212, #3875, #8699, #12161, #2852, #7675, #14520, #6097, #5214, #13489, #13564, #12390, #1493, #8619, #2773, #4983, #5060, #71, #4910, #3713, #2535, #6331, #7365, #9799, #11143, #298, #5137, #7595 ),
 .UNSPECIFIED., .F., .F.,
 ( 4, 2, 2, 2, 2, 2, 2, 2, 2, 2, 2, 2, 2, 2, 2, 2, 2, 2, 2, 2, 2, 4 ),
 ( 0.000000000000000000, 0.01154246058414762008, 0.06319472280952896648, 0.1156547325041140800, 0.1678637871092111822, 0.2189476930995808979, 0.2714221776790743945, 0.3227197530690046334, 0.3747274728241424824, 0.4267432521036158555, 0.4780248536244998681, 0.5305055628088307662, 0.5815973485975094448, 0.6337991395759137170, 0.6855599279679012170, 0.7371634071600560167, 0.7894711232639126663, 0.8405207634104210346, 0.8929453349049019106, 0.9452650328228678900, 0.9965476795071586125, 1.000000000000000000 ),
 .UNSPECIFIED. ) ;
#15546=EDGE_LOOP ( 'NONE', ( #1186, #10065, #14704, #15443 ) ) ;
#15557=CARTESIAN_POINT ( 'NONE',  ( 194.8335778941103626, 33.83376941343732369, -4.128887708184892702 ) ) ;
#15558=AXIS2_PLACEMENT_3D ( 'NONE', #12323, #13815, #11156 ) ;
#15560=DIRECTION ( 'NONE',  ( -0.000000000000000000, -1.000000000000000000, -0.000000000000000000 ) ) ;
#15563=CIRCLE ( 'NONE', #6014, 6.299128011492294732 ) ;
#15568=CARTESIAN_POINT ( 'NONE',  ( 201.3910773252651438, 49.55986643532389735, -5.240523689774838623 ) ) ;
#15570=DIRECTION ( 'NONE',  ( 0.5602235199536450549, 0.8138631617988982825, 0.1541958545404128744 ) ) ;
#15575=EDGE_CURVE ( 'NONE', #14187, #8873, #14310, .T. ) ;
#15586=CIRCLE ( 'NONE', #7798, 20.41351791792154913 ) ;
#15591=CARTESIAN_POINT ( 'NONE',  ( 171.7208925888976978, 62.57671370024034729, -0.9107274384406883749 ) ) ;
#15611=APPLICATION_CONTEXT ( 'automotive_design' ) ;
ENDSEC;
END-ISO-10303-21;
